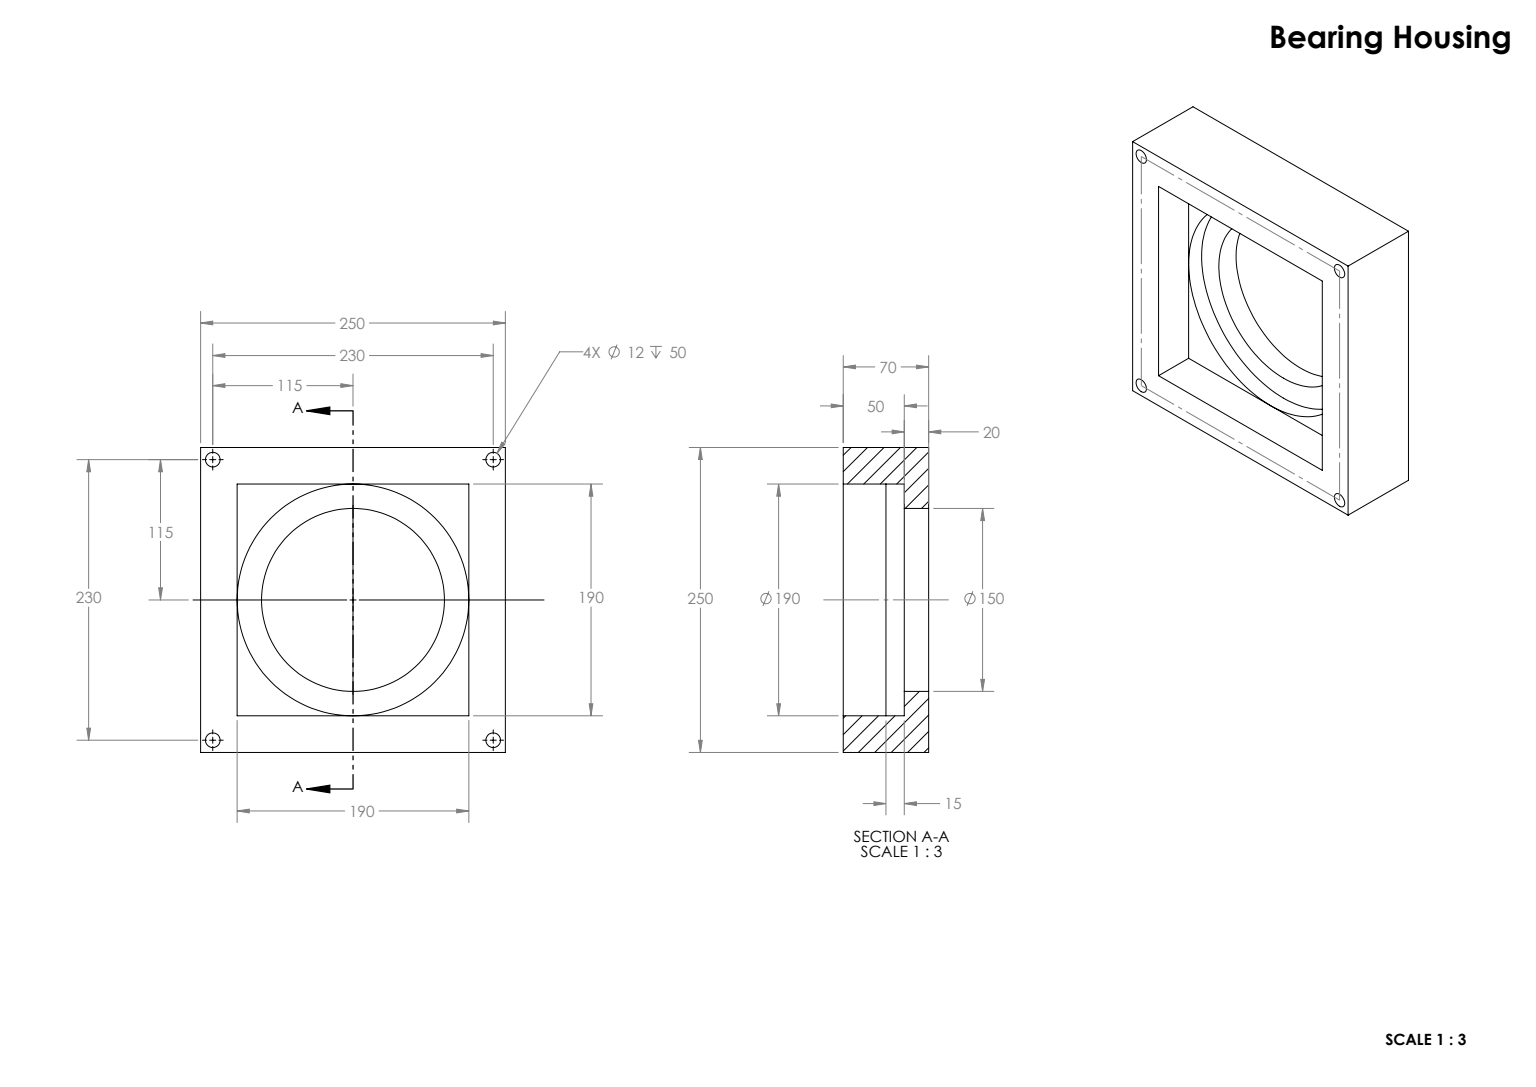
ISO-10303-21;
HEADER;
FILE_DESCRIPTION (('STEP AP214'),
    '1' );
FILE_NAME ('Bearing Housing.step',
    '2026-10-28T15:55:38',
    ( '' ),
    ( '' ),
    'SwSTEP 2.0',
    'SolidWorks 2025',
    '' );
FILE_SCHEMA (( 'AUTOMOTIVE_DESIGN' ));
ENDSEC;

DATA;
#4=LINE ( 'NONE', #7838, #2304 ) ;
#11=DIRECTION ( 'NONE',  ( 1.000000000000000000, 0.000000000000000000, 0.000000000000000000 ) ) ;
#20=DIRECTION ( 'NONE',  ( 0.000000000000000000, 0.000000000000000000, 1.000000000000000000 ) ) ;
#23=CARTESIAN_POINT ( 'NONE',  ( 0.000000000000000000, 0.000000000000000000, 20.00000000000000355 ) ) ;
#31=EDGE_CURVE ( 'NONE', #4444, #7082, #3495, .T. ) ;
#34=DIRECTION ( 'NONE',  ( -0.8571673007021112234, 1.049727191138617340E-16, 0.5150380749100560429 ) ) ;
#38=AXIS2_PLACEMENT_3D ( 'NONE', #602, #6938, #1699 ) ;
#44=ORIENTED_EDGE ( 'NONE', *, *, #3394, .T. ) ;
#47=AXIS2_PLACEMENT_3D ( 'NONE', #5788, #2622, #1664 ) ;
#52=ADVANCED_FACE ( 'NONE', ( #2135 ), #3528, .F. ) ;
#80=LINE ( 'NONE', #6946, #4020 ) ;
#96=ORIENTED_EDGE ( 'NONE', *, *, #4997, .F. ) ;
#128=DIRECTION ( 'NONE',  ( 1.000000000000000000, 0.000000000000000000, 0.000000000000000000 ) ) ;
#148=AXIS2_PLACEMENT_3D ( 'NONE', #811, #7440, #4371 ) ;
#150=ORIENTED_EDGE ( 'NONE', *, *, #4776, .F. ) ;
#160=CARTESIAN_POINT ( 'NONE',  ( -125.0000000000000000, -125.0000000000000284, 70.00000000000000000 ) ) ;
#167=VERTEX_POINT ( 'NONE', #2262 ) ;
#169=ORIENTED_EDGE ( 'NONE', *, *, #6813, .T. ) ;
#172=DIRECTION ( 'NONE',  ( 0.8571673007021112234, 0.000000000000000000, 0.5150380749100560429 ) ) ;
#194=LINE ( 'NONE', #930, #7129 ) ;
#195=DIRECTION ( 'NONE',  ( 0.8571673007021112234, 0.000000000000000000, 0.5150380749100560429 ) ) ;
#204=ADVANCED_FACE ( 'NONE', ( #6375 ), #5709, .F. ) ;
#215=VECTOR ( 'NONE', #34, 1000.000000000000000 ) ;
#226=EDGE_CURVE ( 'NONE', #3065, #4648, #8287, .T. ) ;
#228=DIRECTION ( 'NONE',  ( -0.000000000000000000, -0.000000000000000000, 1.000000000000000000 ) ) ;
#230=DIRECTION ( 'NONE',  ( 1.000000000000000000, 0.000000000000000000, 0.000000000000000000 ) ) ;
#251=DIRECTION ( 'NONE',  ( 1.000000000000000000, 0.000000000000000000, 0.000000000000000000 ) ) ;
#269=CARTESIAN_POINT ( 'NONE',  ( 121.0000000000000284, -115.0000000000000000, 20.00000000000000355 ) ) ;
#294=ORIENTED_EDGE ( 'NONE', *, *, #3089, .F. ) ;
#302=( NAMED_UNIT ( * ) SI_UNIT ( $, .STERADIAN. ) SOLID_ANGLE_UNIT ( ) );
#311=PLANE ( 'NONE',  #4412 ) ;
#313=DIRECTION ( 'NONE',  ( -0.000000000000000000, -0.000000000000000000, 1.000000000000000000 ) ) ;
#318=CARTESIAN_POINT ( 'NONE',  ( 115.0000000000000284, -115.0000000000000000, 20.00000000000000355 ) ) ;
#321=VERTEX_POINT ( 'NONE', #4199 ) ;
#324=CYLINDRICAL_SURFACE ( 'NONE', #1742, 5.999999999999991118 ) ;
#338=AXIS2_PLACEMENT_3D ( 'NONE', #4056, #6518, #5262 ) ;
#357=ORIENTED_EDGE ( 'NONE', *, *, #7077, .F. ) ;
#363=CARTESIAN_POINT ( 'NONE',  ( 115.0000000000000000, 115.0000000000000000, 70.00000000000000000 ) ) ;
#389=DIRECTION ( 'NONE',  ( -0.000000000000000000, -0.000000000000000000, 1.000000000000000000 ) ) ;
#390=AXIS2_PLACEMENT_3D ( 'NONE', #5966, #1418, #2752 ) ;
#393=ADVANCED_FACE ( 'NONE', ( #3838 ), #3197, .T. ) ;
#394=DIRECTION ( 'NONE',  ( 0.000000000000000000, 0.000000000000000000, 1.000000000000000000 ) ) ;
#396=EDGE_CURVE ( 'NONE', #4375, #2961, #3878, .T. ) ;
#398=DIRECTION ( 'NONE',  ( 0.000000000000000000, 0.000000000000000000, 1.000000000000000000 ) ) ;
#399=ORIENTED_EDGE ( 'NONE', *, *, #419, .F. ) ;
#400=LINE ( 'NONE', #8042, #670 ) ;
#405=ORIENTED_EDGE ( 'NONE', *, *, #8301, .F. ) ;
#409=ORIENTED_EDGE ( 'NONE', *, *, #5829, .F. ) ;
#410=FACE_OUTER_BOUND ( 'NONE', #2022, .T. ) ;
#419=EDGE_CURVE ( 'NONE', #3125, #7541, #3274, .T. ) ;
#421=VECTOR ( 'NONE', #7428, 1000.000000000000000 ) ;
#431=VERTEX_POINT ( 'NONE', #681 ) ;
#445=DIRECTION ( 'NONE',  ( 0.000000000000000000, 0.000000000000000000, 1.000000000000000000 ) ) ;
#451=DIRECTION ( 'NONE',  ( -1.000000000000000000, 0.000000000000000000, -0.000000000000000000 ) ) ;
#478=EDGE_LOOP ( 'NONE', ( #2078, #3169, #678, #44 ) ) ;
#481=ORIENTED_EDGE ( 'NONE', *, *, #4733, .F. ) ;
#485=EDGE_LOOP ( 'NONE', ( #1792, #6365 ) ) ;
#488=( GEOMETRIC_REPRESENTATION_CONTEXT ( 3 ) GLOBAL_UNCERTAINTY_ASSIGNED_CONTEXT ( ( #3697 ) ) GLOBAL_UNIT_ASSIGNED_CONTEXT ( ( #6897, #8033, #302 ) ) REPRESENTATION_CONTEXT ( 'NONE', 'WORKASPACE' ) );
#492=ORIENTED_EDGE ( 'NONE', *, *, #5575, .T. ) ;
#519=CONICAL_SURFACE ( 'NONE', #3466, 5.999999999999991118, 1.029744258676652313 ) ;
#520=LINE ( 'NONE', #6379, #1616 ) ;
#529=ADVANCED_FACE ( 'NONE', ( #545, #1858, #8136, #5692, #587, #3655 ), #2328, .F. ) ;
#530=EDGE_CURVE ( 'NONE', #7082, #2571, #3537, .T. ) ;
#545=FACE_BOUND ( 'NONE', #6221, .T. ) ;
#555=CARTESIAN_POINT ( 'NONE',  ( -94.99999999999997158, -95.00000000000008527, 35.00000000000000000 ) ) ;
#557=PRODUCT_DEFINITION ( 'UNKNOWN', '', #4198, #6779 ) ;
#560=ADVANCED_FACE ( 'NONE', ( #3064 ), #3869, .F. ) ;
#567=ORIENTED_EDGE ( 'NONE', *, *, #3332, .F. ) ;
#587=FACE_OUTER_BOUND ( 'NONE', #4365, .T. ) ;
#588=EDGE_LOOP ( 'NONE', ( #4360, #4935, #2316, #3157, #5452 ) ) ;
#590=DIRECTION ( 'NONE',  ( -0.000000000000000000, -0.000000000000000000, -1.000000000000000000 ) ) ;
#594=ADVANCED_BREP_SHAPE_REPRESENTATION ( '', ( #3512, #1299 ), #2770 ) ;
#599=ORIENTED_EDGE ( 'NONE', *, *, #1346, .F. ) ;
#602=CARTESIAN_POINT ( 'NONE',  ( 0.000000000000000000, 0.000000000000000000, 20.00000000000000355 ) ) ;
#606=ADVANCED_FACE ( 'NONE', ( #7629 ), #2357, .F. ) ;
#608=EDGE_LOOP ( 'NONE', ( #5995, #599, #5529 ) ) ;
#613=CARTESIAN_POINT ( 'NONE',  ( 0.000000000000000000, 0.000000000000000000, 35.00000000000000000 ) ) ;
#621=LINE ( 'NONE', #7198, #5046 ) ;
#631=ORIENTED_EDGE ( 'NONE', *, *, #7077, .T. ) ;
#635=DIRECTION ( 'NONE',  ( -0.000000000000000000, -0.000000000000000000, -1.000000000000000000 ) ) ;
#646=AXIS2_PLACEMENT_3D ( 'NONE', #788, #6612, #832 ) ;
#647=LINE ( 'NONE', #3893, #4845 ) ;
#663=DIRECTION ( 'NONE',  ( 1.000000000000000000, 0.000000000000000000, 0.000000000000000000 ) ) ;
#670=VECTOR ( 'NONE', #4828, 1000.000000000000000 ) ;
#673=CARTESIAN_POINT ( 'NONE',  ( 115.0000000000000284, -115.0000000000000000, 20.00000000000000355 ) ) ;
#675=DIRECTION ( 'NONE',  ( 0.000000000000000000, -1.000000000000000000, 0.000000000000000000 ) ) ;
#678=ORIENTED_EDGE ( 'NONE', *, *, #2723, .T. ) ;
#681=CARTESIAN_POINT ( 'NONE',  ( 95.00000000000000000, 95.00000000000008527, 35.00000000000000000 ) ) ;
#682=LINE ( 'NONE', #2005, #3999 ) ;
#704=DIRECTION ( 'NONE',  ( -0.000000000000000000, -0.000000000000000000, -1.000000000000000000 ) ) ;
#709=CARTESIAN_POINT ( 'NONE',  ( 0.000000000000000000, 0.000000000000000000, 35.00000000000000000 ) ) ;
#738=VECTOR ( 'NONE', #3922, 1000.000000000000000 ) ;
#749=FACE_OUTER_BOUND ( 'NONE', #4846, .T. ) ;
#750=ORIENTED_EDGE ( 'NONE', *, *, #3807, .F. ) ;
#761=CARTESIAN_POINT ( 'NONE',  ( -121.0000000000000284, -115.0000000000000000, 70.00000000000000000 ) ) ;
#765=CIRCLE ( 'NONE', #5482, 5.999999999999991118 ) ;
#770=DIRECTION ( 'NONE',  ( -0.8571673007021112234, 1.049727191138617340E-16, 0.5150380749100560429 ) ) ;
#783=VECTOR ( 'NONE', #770, 1000.000000000000000 ) ;
#784=LINE ( 'NONE', #7845, #3091 ) ;
#788=CARTESIAN_POINT ( 'NONE',  ( -125.0000000000000000, -125.0000000000000284, 70.00000000000000000 ) ) ;
#811=CARTESIAN_POINT ( 'NONE',  ( -115.0000000000000000, 115.0000000000000000, 70.00000000000000000 ) ) ;
#824=ADVANCED_FACE ( 'NONE', ( #6135 ), #881, .F. ) ;
#832=DIRECTION ( 'NONE',  ( 0.000000000000000000, 0.000000000000000000, -1.000000000000000000 ) ) ;
#840=EDGE_CURVE ( 'NONE', #4413, #3125, #621, .T. ) ;
#845=ORIENTED_EDGE ( 'NONE', *, *, #5575, .F. ) ;
#858=AXIS2_PLACEMENT_3D ( 'NONE', #1793, #3675, #1748 ) ;
#865=CARTESIAN_POINT ( 'NONE',  ( -125.0000000000000000, 125.0000000000000284, 70.00000000000000000 ) ) ;
#867=CARTESIAN_POINT ( 'NONE',  ( 125.0000000000000000, -125.0000000000000284, 70.00000000000000000 ) ) ;
#868=LINE ( 'NONE', #4741, #4236 ) ;
#881=CYLINDRICAL_SURFACE ( 'NONE', #5727, 95.00000000000008527 ) ;
#887=ORIENTED_EDGE ( 'NONE', *, *, #4997, .T. ) ;
#894=DIRECTION ( 'NONE',  ( 0.000000000000000000, -0.000000000000000000, -1.000000000000000000 ) ) ;
#899=ORIENTED_EDGE ( 'NONE', *, *, #2632, .F. ) ;
#904=CARTESIAN_POINT ( 'NONE',  ( 121.0000000000000284, -115.0000000000000000, 20.00000000000000355 ) ) ;
#910=FACE_OUTER_BOUND ( 'NONE', #7824, .T. ) ;
#930=CARTESIAN_POINT ( 'NONE',  ( -94.99999999999997158, -95.00000000000008527, 70.00000000000000000 ) ) ;
#946=EDGE_LOOP ( 'NONE', ( #1027, #5506, #399, #5076 ) ) ;
#948=FACE_OUTER_BOUND ( 'NONE', #4156, .T. ) ;
#984=VERTEX_POINT ( 'NONE', #1023 ) ;
#985=CARTESIAN_POINT ( 'NONE',  ( -115.0000000000000000, 115.0000000000000000, 20.00000000000000355 ) ) ;
#999=DIRECTION ( 'NONE',  ( -1.000000000000000000, -2.921639538487254261E-16, 0.000000000000000000 ) ) ;
#1002=DIRECTION ( 'NONE',  ( 1.000000000000000000, 0.000000000000000000, 0.000000000000000000 ) ) ;
#1003=ORIENTED_EDGE ( 'NONE', *, *, #8301, .T. ) ;
#1015=EDGE_CURVE ( 'NONE', #7541, #321, #4599, .T. ) ;
#1023=CARTESIAN_POINT ( 'NONE',  ( 0.000000000000000000, 95.00000000000008527, 35.00000000000000000 ) ) ;
#1027=ORIENTED_EDGE ( 'NONE', *, *, #7821, .F. ) ;
#1030=VECTOR ( 'NONE', #5810, 1000.000000000000000 ) ;
#1045=FACE_OUTER_BOUND ( 'NONE', #5118, .T. ) ;
#1071=CARTESIAN_POINT ( 'NONE',  ( 115.0000000000000142, -115.0000000000000000, 16.39483628583463570 ) ) ;
#1074=DIRECTION ( 'NONE',  ( 0.000000000000000000, 0.000000000000000000, 1.000000000000000000 ) ) ;
#1085=LINE ( 'NONE', #1631, #4556 ) ;
#1086=CIRCLE ( 'NONE', #5804, 5.999999999999991118 ) ;
#1090=DIRECTION ( 'NONE',  ( -0.000000000000000000, -0.000000000000000000, 1.000000000000000000 ) ) ;
#1096=ORIENTED_EDGE ( 'NONE', *, *, #5028, .T. ) ;
#1097=CARTESIAN_POINT ( 'NONE',  ( -109.0000000000000426, -115.0000000000000000, 20.00000000000000355 ) ) ;
#1102=ORIENTED_EDGE ( 'NONE', *, *, #8208, .F. ) ;
#1111=CARTESIAN_POINT ( 'NONE',  ( -95.00000000000008527, 1.163414459189986590E-14, 20.00000000000000355 ) ) ;
#1137=EDGE_LOOP ( 'NONE', ( #6698, #6760, #1494 ) ) ;
#1140=ORIENTED_EDGE ( 'NONE', *, *, #7652, .T. ) ;
#1142=DIRECTION ( 'NONE',  ( -0.000000000000000000, -0.000000000000000000, 1.000000000000000000 ) ) ;
#1162=LINE ( 'NONE', #2390, #1897 ) ;
#1173=CIRCLE ( 'NONE', #5753, 5.999999999999991118 ) ;
#1182=FACE_OUTER_BOUND ( 'NONE', #1137, .T. ) ;
#1188=EDGE_CURVE ( 'NONE', #4648, #3065, #3811, .T. ) ;
#1194=DIRECTION ( 'NONE',  ( -0.000000000000000000, -0.000000000000000000, 1.000000000000000000 ) ) ;
#1197=EDGE_CURVE ( 'NONE', #4172, #3595, #4328, .T. ) ;
#1226=DIRECTION ( 'NONE',  ( -0.000000000000000000, -0.000000000000000000, 1.000000000000000000 ) ) ;
#1227=PLANE ( 'NONE',  #7361 ) ;
#1245=EDGE_CURVE ( 'NONE', #6477, #2906, #6366, .T. ) ;
#1253=DIRECTION ( 'NONE',  ( 0.000000000000000000, 0.000000000000000000, -1.000000000000000000 ) ) ;
#1267=FACE_OUTER_BOUND ( 'NONE', #4745, .T. ) ;
#1276=VECTOR ( 'NONE', #1311, 1000.000000000000000 ) ;
#1277=VERTEX_POINT ( 'NONE', #7565 ) ;
#1280=DIRECTION ( 'NONE',  ( -0.000000000000000000, -0.000000000000000000, 1.000000000000000000 ) ) ;
#1286=EDGE_LOOP ( 'NONE', ( #1102, #7331, #2428 ) ) ;
#1287=ORIENTED_EDGE ( 'NONE', *, *, #6688, .F. ) ;
#1290=DIRECTION ( 'NONE',  ( -0.000000000000000000, -0.000000000000000000, 1.000000000000000000 ) ) ;
#1293=CARTESIAN_POINT ( 'NONE',  ( -115.0000000000000000, 115.0000000000000000, 70.00000000000000000 ) ) ;
#1299=AXIS2_PLACEMENT_3D ( 'NONE', #5884, #1507, #5927 ) ;
#1310=ORIENTED_EDGE ( 'NONE', *, *, #2278, .T. ) ;
#1311=DIRECTION ( 'NONE',  ( 1.000000000000000000, -0.000000000000000000, -0.000000000000000000 ) ) ;
#1346=EDGE_CURVE ( 'NONE', #4671, #5876, #4609, .T. ) ;
#1371=DIRECTION ( 'NONE',  ( -1.000000000000000000, -2.921639538487254261E-16, 0.000000000000000000 ) ) ;
#1389=LINE ( 'NONE', #5624, #1594 ) ;
#1396=ORIENTED_EDGE ( 'NONE', *, *, #3184, .T. ) ;
#1409=DIRECTION ( 'NONE',  ( -0.000000000000000000, -0.000000000000000000, 1.000000000000000000 ) ) ;
#1414=ORIENTED_EDGE ( 'NONE', *, *, #8095, .F. ) ;
#1418=DIRECTION ( 'NONE',  ( -0.000000000000000000, -0.000000000000000000, 1.000000000000000000 ) ) ;
#1421=FACE_OUTER_BOUND ( 'NONE', #1500, .T. ) ;
#1423=DIRECTION ( 'NONE',  ( 1.000000000000000000, 0.000000000000000000, 0.000000000000000000 ) ) ;
#1452=ORIENTED_EDGE ( 'NONE', *, *, #5795, .T. ) ;
#1455=CARTESIAN_POINT ( 'NONE',  ( 95.00000000000008527, 1.387778780781445991E-14, 35.00000000000000000 ) ) ;
#1456=ADVANCED_FACE ( 'NONE', ( #910 ), #8038, .F. ) ;
#1466=DIRECTION ( 'NONE',  ( 1.000000000000000000, 0.000000000000000000, 0.000000000000000000 ) ) ;
#1478=EDGE_LOOP ( 'NONE', ( #2814, #4335, #7683, #8119 ) ) ;
#1484=EDGE_CURVE ( 'NONE', #6102, #3725, #5831, .T. ) ;
#1494=ORIENTED_EDGE ( 'NONE', *, *, #530, .T. ) ;
#1497=ADVANCED_FACE ( 'NONE', ( #5339 ), #2472, .F. ) ;
#1500=EDGE_LOOP ( 'NONE', ( #2987, #3974, #150, #5372 ) ) ;
#1507=DIRECTION ( 'NONE',  ( 0.000000000000000000, 0.000000000000000000, 1.000000000000000000 ) ) ;
#1509=LINE ( 'NONE', #4179, #8200 ) ;
#1517=CARTESIAN_POINT ( 'NONE',  ( 115.0000000000000284, -115.0000000000000000, 70.00000000000000000 ) ) ;
#1526=CARTESIAN_POINT ( 'NONE',  ( 0.000000000000000000, 0.000000000000000000, 20.00000000000000355 ) ) ;
#1528=DIRECTION ( 'NONE',  ( 0.000000000000000000, 0.000000000000000000, -1.000000000000000000 ) ) ;
#1561=CARTESIAN_POINT ( 'NONE',  ( 109.0000000000000426, -115.0000000000000000, 70.00000000000000000 ) ) ;
#1564=EDGE_CURVE ( 'NONE', #2906, #6477, #2478, .T. ) ;
#1569=VECTOR ( 'NONE', #8345, 1000.000000000000000 ) ;
#1570=LINE ( 'NONE', #160, #5897 ) ;
#1577=ORIENTED_EDGE ( 'NONE', *, *, #2769, .T. ) ;
#1583=CIRCLE ( 'NONE', #5077, 75.00000000000001421 ) ;
#1594=VECTOR ( 'NONE', #7128, 1000.000000000000000 ) ;
#1600=ADVANCED_FACE ( 'NONE', ( #3544, #6125 ), #5512, .T. ) ;
#1616=VECTOR ( 'NONE', #7534, 1000.000000000000000 ) ;
#1631=CARTESIAN_POINT ( 'NONE',  ( 95.00000000000002842, -95.00000000000002842, 35.00000000000000000 ) ) ;
#1639=CIRCLE ( 'NONE', #6351, 75.00000000000001421 ) ;
#1664=DIRECTION ( 'NONE',  ( -1.000000000000000000, -2.921639538487254261E-16, 0.000000000000000000 ) ) ;
#1667=CLOSED_SHELL ( 'NONE', ( #2679, #1880, #7336, #2122, #6642, #3883, #8031, #3707, #824, #6804, #606, #5668, #52, #4927, #1815, #5762, #393, #2091, #529, #4372, #8145, #2776, #6343, #204, #3859, #1600, #7114, #6811, #2441, #3318, #560, #4099, #1456, #1497, #6513 ) ) ;
#1668=CARTESIAN_POINT ( 'NONE',  ( -94.99999999999997158, -95.00000000000008527, 70.00000000000000000 ) ) ;
#1670=DIRECTION ( 'NONE',  ( 0.000000000000000000, 0.000000000000000000, -1.000000000000000000 ) ) ;
#1684=ORIENTED_EDGE ( 'NONE', *, *, #2388, .T. ) ;
#1699=DIRECTION ( 'NONE',  ( 1.000000000000000000, 0.000000000000000000, 0.000000000000000000 ) ) ;
#1734=ORIENTED_EDGE ( 'NONE', *, *, #5795, .F. ) ;
#1735=DIRECTION ( 'NONE',  ( -0.000000000000000000, -0.000000000000000000, -1.000000000000000000 ) ) ;
#1742=AXIS2_PLACEMENT_3D ( 'NONE', #2367, #4918, #4885 ) ;
#1748=DIRECTION ( 'NONE',  ( 0.000000000000000000, 0.000000000000000000, 1.000000000000000000 ) ) ;
#1763=CARTESIAN_POINT ( 'NONE',  ( -115.0000000000000000, 115.0000000000000000, 70.00000000000000000 ) ) ;
#1766=VECTOR ( 'NONE', #3795, 1000.000000000000000 ) ;
#1768=ORIENTED_EDGE ( 'NONE', *, *, #4192, .T. ) ;
#1773=ORIENTED_EDGE ( 'NONE', *, *, #396, .T. ) ;
#1783=EDGE_LOOP ( 'NONE', ( #8289, #4269, #7405, #2363 ) ) ;
#1785=CYLINDRICAL_SURFACE ( 'NONE', #1873, 75.00000000000001421 ) ;
#1792=ORIENTED_EDGE ( 'NONE', *, *, #3763, .F. ) ;
#1793=CARTESIAN_POINT ( 'NONE',  ( 125.0000000000000000, -125.0000000000000284, 70.00000000000000000 ) ) ;
#1802=CARTESIAN_POINT ( 'NONE',  ( 95.00000000000000000, 95.00000000000008527, 70.00000000000000000 ) ) ;
#1815=ADVANCED_FACE ( 'NONE', ( #7307 ), #4081, .T. ) ;
#1820=EDGE_LOOP ( 'NONE', ( #4840, #1734, #409 ) ) ;
#1850=LINE ( 'NONE', #2451, #2663 ) ;
#1852=ORIENTED_EDGE ( 'NONE', *, *, #7492, .T. ) ;
#1854=AXIS2_PLACEMENT_3D ( 'NONE', #4858, #5664, #6078 ) ;
#1858=FACE_BOUND ( 'NONE', #485, .T. ) ;
#1866=EDGE_CURVE ( 'NONE', #6494, #167, #4693, .T. ) ;
#1873=AXIS2_PLACEMENT_3D ( 'NONE', #7567, #1735, #7517 ) ;
#1880=ADVANCED_FACE ( 'NONE', ( #948 ), #2153, .F. ) ;
#1897=VECTOR ( 'NONE', #1280, 1000.000000000000000 ) ;
#1906=ORIENTED_EDGE ( 'NONE', *, *, #2484, .T. ) ;
#1940=CARTESIAN_POINT ( 'NONE',  ( 115.0000000000000284, -115.0000000000000000, 70.00000000000000000 ) ) ;
#1949=ORIENTED_EDGE ( 'NONE', *, *, #8105, .F. ) ;
#1979=FACE_OUTER_BOUND ( 'NONE', #608, .T. ) ;
#1994=ORIENTED_EDGE ( 'NONE', *, *, #2474, .T. ) ;
#2003=MECHANICAL_DESIGN_GEOMETRIC_PRESENTATION_REPRESENTATION('',(#5880),#488);
#2005=CARTESIAN_POINT ( 'NONE',  ( 121.0000000000000284, -115.0000000000000000, 70.00000000000000000 ) ) ;
#2010=AXIS2_PLACEMENT_3D ( 'NONE', #7360, #7954, #8028 ) ;
#2015=CARTESIAN_POINT ( 'NONE',  ( 95.00000000000002842, -95.00000000000002842, 70.00000000000000000 ) ) ;
#2022=EDGE_LOOP ( 'NONE', ( #6636, #1140, #3559, #3514 ) ) ;
#2052=ORIENTED_EDGE ( 'NONE', *, *, #6603, .T. ) ;
#2064=PRODUCT_DEFINITION_SHAPE ( 'NONE', 'NONE',  #557 ) ;
#2078=ORIENTED_EDGE ( 'NONE', *, *, #8225, .F. ) ;
#2085=AXIS2_PLACEMENT_3D ( 'NONE', #5602, #445, #663 ) ;
#2091=ADVANCED_FACE ( 'NONE', ( #2215 ), #6199, .T. ) ;
#2093=CARTESIAN_POINT ( 'NONE',  ( 125.0000000000000000, -125.0000000000000284, 70.00000000000000000 ) ) ;
#2107=ORIENTED_EDGE ( 'NONE', *, *, #1564, .T. ) ;
#2122=ADVANCED_FACE ( 'NONE', ( #6834 ), #5407, .F. ) ;
#2135=FACE_OUTER_BOUND ( 'NONE', #1820, .T. ) ;
#2147=SHAPE_REPRESENTATION_RELATIONSHIP ( 'NONE' , 'NONE' ,  #2264, #594 ) ;
#2153=CONICAL_SURFACE ( 'NONE', #6444, 5.999999999999991118, 1.029744258676652313 ) ;
#2159=VECTOR ( 'NONE', #4968, 1000.000000000000000 ) ;
#2161=ORIENTED_EDGE ( 'NONE', *, *, #3332, .T. ) ;
#2165=ORIENTED_EDGE ( 'NONE', *, *, #1564, .F. ) ;
#2181=CARTESIAN_POINT ( 'NONE',  ( 115.0000000000000284, -115.0000000000000000, 20.00000000000000355 ) ) ;
#2183=EDGE_CURVE ( 'NONE', #2571, #5439, #5014, .T. ) ;
#2205=LINE ( 'NONE', #5561, #421 ) ;
#2208=UNCERTAINTY_MEASURE_WITH_UNIT (LENGTH_MEASURE( 1.000000000000000082E-05 ), #5967, 'distance_accuracy_value', 'NONE');
#2212=CYLINDRICAL_SURFACE ( 'NONE', #3779, 5.999999999999991118 ) ;
#2215=FACE_OUTER_BOUND ( 'NONE', #4169, .T. ) ;
#2221=LINE ( 'NONE', #4002, #783 ) ;
#2243=CARTESIAN_POINT ( 'NONE',  ( 0.000000000000000000, 0.000000000000000000, 35.00000000000000000 ) ) ;
#2258=ORIENTED_EDGE ( 'NONE', *, *, #2769, .F. ) ;
#2262=CARTESIAN_POINT ( 'NONE',  ( -109.0000000000000426, -115.0000000000000000, 70.00000000000000000 ) ) ;
#2264=SHAPE_REPRESENTATION ( 'Bearing Housing', ( #1299 ), #2770 ) ;
#2266=AXIS2_PLACEMENT_3D ( 'NONE', #613, #1253, #7661 ) ;
#2278=EDGE_CURVE ( 'NONE', #3595, #167, #7171, .T. ) ;
#2295=DIRECTION ( 'NONE',  ( 1.460819769243626145E-16, -1.000000000000000000, 0.000000000000000000 ) ) ;
#2304=VECTOR ( 'NONE', #7793, 1000.000000000000000 ) ;
#2313=DIRECTION ( 'NONE',  ( 1.000000000000000000, 0.000000000000000000, -0.000000000000000000 ) ) ;
#2316=ORIENTED_EDGE ( 'NONE', *, *, #7896, .T. ) ;
#2317=FACE_OUTER_BOUND ( 'NONE', #4232, .T. ) ;
#2318=DIRECTION ( 'NONE',  ( 1.000000000000000000, 0.000000000000000000, 0.000000000000000000 ) ) ;
#2328=PLANE ( 'NONE',  #7482 ) ;
#2340=DIRECTION ( 'NONE',  ( -0.000000000000000000, -0.000000000000000000, 1.000000000000000000 ) ) ;
#2341=AXIS2_PLACEMENT_3D ( 'NONE', #1763, #7458, #3682 ) ;
#2344=ORIENTED_EDGE ( 'NONE', *, *, #7429, .F. ) ;
#2357=PLANE ( 'NONE',  #2368 ) ;
#2360=DIRECTION ( 'NONE',  ( -0.000000000000000000, -0.000000000000000000, 1.000000000000000000 ) ) ;
#2363=ORIENTED_EDGE ( 'NONE', *, *, #5060, .T. ) ;
#2367=CARTESIAN_POINT ( 'NONE',  ( -115.0000000000000284, -115.0000000000000000, 70.00000000000000000 ) ) ;
#2368=AXIS2_PLACEMENT_3D ( 'NONE', #2922, #1670, #8264 ) ;
#2388=EDGE_CURVE ( 'NONE', #7988, #7828, #2205, .T. ) ;
#2390=CARTESIAN_POINT ( 'NONE',  ( -121.0000000000000284, -115.0000000000000000, 70.00000000000000000 ) ) ;
#2400=EDGE_LOOP ( 'NONE', ( #4395, #3990 ) ) ;
#2402=DIRECTION ( 'NONE',  ( -0.000000000000000000, -0.000000000000000000, 1.000000000000000000 ) ) ;
#2428=ORIENTED_EDGE ( 'NONE', *, *, #1484, .T. ) ;
#2439=ORIENTED_EDGE ( 'NONE', *, *, #7821, .T. ) ;
#2441=ADVANCED_FACE ( 'NONE', ( #1045 ), #7338, .F. ) ;
#2443=CARTESIAN_POINT ( 'NONE',  ( -94.99999999999997158, -95.00000000000008527, 35.00000000000000000 ) ) ;
#2447=CARTESIAN_POINT ( 'NONE',  ( 109.0000000000000142, 115.0000000000000000, 70.00000000000000000 ) ) ;
#2451=CARTESIAN_POINT ( 'NONE',  ( 95.00000000000002842, -95.00000000000002842, 70.00000000000000000 ) ) ;
#2459=DIRECTION ( 'NONE',  ( -0.000000000000000000, -0.000000000000000000, 1.000000000000000000 ) ) ;
#2469=EDGE_LOOP ( 'NONE', ( #2258, #6415 ) ) ;
#2472=CONICAL_SURFACE ( 'NONE', #3513, 5.999999999999991118, 1.029744258676652313 ) ;
#2474=EDGE_CURVE ( 'NONE', #2571, #7082, #3245, .T. ) ;
#2478=CIRCLE ( 'NONE', #2341, 5.999999999999991118 ) ;
#2484=EDGE_CURVE ( 'NONE', #5937, #3656, #1639, .T. ) ;
#2489=CARTESIAN_POINT ( 'NONE',  ( 109.0000000000000426, -115.0000000000000000, 20.00000000000000355 ) ) ;
#2494=CARTESIAN_POINT ( 'NONE',  ( 0.000000000000000000, 0.000000000000000000, 70.00000000000000000 ) ) ;
#2497=DIRECTION ( 'NONE',  ( -0.000000000000000000, -0.000000000000000000, 1.000000000000000000 ) ) ;
#2499=PRODUCT_CONTEXT ( 'NONE', #5106, 'mechanical' ) ;
#2516=VECTOR ( 'NONE', #6500, 1000.000000000000000 ) ;
#2530=CONICAL_SURFACE ( 'NONE', #3578, 5.999999999999991118, 1.029744258676652313 ) ;
#2547=ORIENTED_EDGE ( 'NONE', *, *, #5060, .F. ) ;
#2553=AXIS2_PLACEMENT_3D ( 'NONE', #709, #3266, #5935 ) ;
#2566=DIRECTION ( 'NONE',  ( -0.000000000000000000, -1.000000000000000000, -0.000000000000000000 ) ) ;
#2571=VERTEX_POINT ( 'NONE', #2489 ) ;
#2589=EDGE_LOOP ( 'NONE', ( #7615, #4290, #6395, #5202 ) ) ;
#2592=ORIENTED_EDGE ( 'NONE', *, *, #2183, .T. ) ;
#2593=AXIS2_PLACEMENT_3D ( 'NONE', #1517, #6742, #230 ) ;
#2611=ORIENTED_EDGE ( 'NONE', *, *, #6278, .T. ) ;
#2612=VERTEX_POINT ( 'NONE', #3108 ) ;
#2622=DIRECTION ( 'NONE',  ( -2.921639538487254261E-16, 1.000000000000000000, 0.000000000000000000 ) ) ;
#2632=EDGE_CURVE ( 'NONE', #7988, #3069, #1850, .T. ) ;
#2659=VECTOR ( 'NONE', #195, 1000.000000000000000 ) ;
#2663=VECTOR ( 'NONE', #3824, 1000.000000000000000 ) ;
#2671=CARTESIAN_POINT ( 'NONE',  ( 75.00000000000001421, 9.184850993605150311E-15, 20.00000000000000355 ) ) ;
#2679=ADVANCED_FACE ( 'NONE', ( #4914 ), #6867, .F. ) ;
#2684=FACE_OUTER_BOUND ( 'NONE', #4430, .T. ) ;
#2687=DIRECTION ( 'NONE',  ( -0.000000000000000000, -0.000000000000000000, 1.000000000000000000 ) ) ;
#2689=ORIENTED_EDGE ( 'NONE', *, *, #7492, .F. ) ;
#2723=EDGE_CURVE ( 'NONE', #3656, #5338, #5303, .T. ) ;
#2752=DIRECTION ( 'NONE',  ( 1.000000000000000000, 0.000000000000000000, 0.000000000000000000 ) ) ;
#2754=DIRECTION ( 'NONE',  ( -1.460819769243625652E-16, 1.000000000000000000, 0.000000000000000000 ) ) ;
#2769=EDGE_CURVE ( 'NONE', #167, #6494, #2792, .T. ) ;
#2770=( GEOMETRIC_REPRESENTATION_CONTEXT ( 3 ) GLOBAL_UNCERTAINTY_ASSIGNED_CONTEXT ( ( #2208 ) ) GLOBAL_UNIT_ASSIGNED_CONTEXT ( ( #5967, #3298, #4614 ) ) REPRESENTATION_CONTEXT ( 'NONE', 'WORKASPACE' ) );
#2774=AXIS2_PLACEMENT_3D ( 'NONE', #2181, #1409, #4730 ) ;
#2776=ADVANCED_FACE ( 'NONE', ( #1421 ), #6566, .F. ) ;
#2792=CIRCLE ( 'NONE', #4539, 5.999999999999991118 ) ;
#2793=FACE_OUTER_BOUND ( 'NONE', #946, .T. ) ;
#2802=CARTESIAN_POINT ( 'NONE',  ( -115.0000000000000142, 115.0000000000000000, 16.39483628583463570 ) ) ;
#2814=ORIENTED_EDGE ( 'NONE', *, *, #2484, .F. ) ;
#2815=EDGE_CURVE ( 'NONE', #2961, #321, #1509, .T. ) ;
#2816=FACE_OUTER_BOUND ( 'NONE', #3661, .T. ) ;
#2831=ORIENTED_EDGE ( 'NONE', *, *, #6813, .F. ) ;
#2833=ORIENTED_EDGE ( 'NONE', *, *, #8208, .T. ) ;
#2849=AXIS2_PLACEMENT_3D ( 'NONE', #5425, #7291, #1466 ) ;
#2854=LINE ( 'NONE', #1097, #2159 ) ;
#2885=DIRECTION ( 'NONE',  ( 1.000000000000000000, 0.000000000000000000, 0.000000000000000000 ) ) ;
#2904=CIRCLE ( 'NONE', #5747, 5.999999999999991118 ) ;
#2906=VERTEX_POINT ( 'NONE', #6731 ) ;
#2908=VECTOR ( 'NONE', #8122, 1000.000000000000000 ) ;
#2922=CARTESIAN_POINT ( 'NONE',  ( 0.000000000000000000, 0.000000000000000000, 35.00000000000000000 ) ) ;
#2927=LINE ( 'NONE', #5519, #4384 ) ;
#2928=ORIENTED_EDGE ( 'NONE', *, *, #2183, .F. ) ;
#2937=AXIS2_PLACEMENT_3D ( 'NONE', #7638, #4399, #5778 ) ;
#2951=AXIS2_PLACEMENT_3D ( 'NONE', #8328, #7050, #5827 ) ;
#2961=VERTEX_POINT ( 'NONE', #7273 ) ;
#2986=CARTESIAN_POINT ( 'NONE',  ( 115.0000000000000000, 115.0000000000000000, 20.00000000000000355 ) ) ;
#2987=ORIENTED_EDGE ( 'NONE', *, *, #840, .T. ) ;
#3032=ORIENTED_EDGE ( 'NONE', *, *, #3319, .F. ) ;
#3049=CARTESIAN_POINT ( 'NONE',  ( -109.0000000000000142, 115.0000000000000000, 20.00000000000000355 ) ) ;
#3064=FACE_OUTER_BOUND ( 'NONE', #4958, .T. ) ;
#3065=VERTEX_POINT ( 'NONE', #1111 ) ;
#3067=FACE_OUTER_BOUND ( 'NONE', #5317, .T. ) ;
#3069=VERTEX_POINT ( 'NONE', #6440 ) ;
#3081=ORIENTED_EDGE ( 'NONE', *, *, #3910, .F. ) ;
#3084=DIRECTION ( 'NONE',  ( -1.000000000000000000, 0.000000000000000000, 0.000000000000000000 ) ) ;
#3089=EDGE_CURVE ( 'NONE', #5894, #5749, #1389, .T. ) ;
#3091=VECTOR ( 'NONE', #3374, 1000.000000000000000 ) ;
#3108=CARTESIAN_POINT ( 'NONE',  ( -95.00000000000000000, 95.00000000000008527, 70.00000000000000000 ) ) ;
#3109=ORIENTED_EDGE ( 'NONE', *, *, #4431, .F. ) ;
#3125=VERTEX_POINT ( 'NONE', #6009 ) ;
#3157=ORIENTED_EDGE ( 'NONE', *, *, #3184, .F. ) ;
#3169=ORIENTED_EDGE ( 'NONE', *, *, #8157, .F. ) ;
#3182=CONICAL_SURFACE ( 'NONE', #1854, 5.999999999999991118, 1.029744258676652313 ) ;
#3184=EDGE_CURVE ( 'NONE', #7934, #6392, #3386, .T. ) ;
#3197=PLANE ( 'NONE',  #47 ) ;
#3204=CARTESIAN_POINT ( 'NONE',  ( -121.0000000000000284, -115.0000000000000000, 20.00000000000000355 ) ) ;
#3211=CARTESIAN_POINT ( 'NONE',  ( -109.0000000000000426, -115.0000000000000000, 20.00000000000000355 ) ) ;
#3214=VECTOR ( 'NONE', #3821, 1000.000000000000000 ) ;
#3216=LINE ( 'NONE', #7674, #6696 ) ;
#3217=LINE ( 'NONE', #4351, #3214 ) ;
#3230=DIRECTION ( 'NONE',  ( 1.000000000000000000, 0.000000000000000000, 0.000000000000000000 ) ) ;
#3233=DIRECTION ( 'NONE',  ( 1.000000000000000000, 0.000000000000000000, 0.000000000000000000 ) ) ;
#3245=CIRCLE ( 'NONE', #5948, 5.999999999999991118 ) ;
#3256=DIRECTION ( 'NONE',  ( -0.000000000000000000, -0.000000000000000000, 1.000000000000000000 ) ) ;
#3257=CARTESIAN_POINT ( 'NONE',  ( -95.00000000000000000, 95.00000000000008527, 35.00000000000000000 ) ) ;
#3266=DIRECTION ( 'NONE',  ( 0.000000000000000000, 0.000000000000000000, -1.000000000000000000 ) ) ;
#3272=VECTOR ( 'NONE', #172, 1000.000000000000000 ) ;
#3274=LINE ( 'NONE', #5145, #1276 ) ;
#3285=CARTESIAN_POINT ( 'NONE',  ( -94.99999999999998579, -1.387778780781444098E-14, 35.00000000000000000 ) ) ;
#3298=( NAMED_UNIT ( * ) PLANE_ANGLE_UNIT ( ) SI_UNIT ( $, .RADIAN. ) );
#3318=ADVANCED_FACE ( 'NONE', ( #6183 ), #6687, .F. ) ;
#3319=EDGE_CURVE ( 'NONE', #4648, #4314, #2927, .T. ) ;
#3326=CARTESIAN_POINT ( 'NONE',  ( -94.99999999999997158, -95.00000000000008527, 70.00000000000000000 ) ) ;
#3332=EDGE_CURVE ( 'NONE', #3595, #4172, #765, .T. ) ;
#3333=EDGE_CURVE ( 'NONE', #6102, #8341, #4871, .T. ) ;
#3374=DIRECTION ( 'NONE',  ( -0.000000000000000000, -0.000000000000000000, 1.000000000000000000 ) ) ;
#3375=EDGE_CURVE ( 'NONE', #5439, #5603, #2904, .T. ) ;
#3386=LINE ( 'NONE', #7297, #4260 ) ;
#3394=EDGE_CURVE ( 'NONE', #5338, #6480, #7645, .T. ) ;
#3402=CARTESIAN_POINT ( 'NONE',  ( -109.0000000000000142, 115.0000000000000000, 70.00000000000000000 ) ) ;
#3426=CARTESIAN_POINT ( 'NONE',  ( 0.000000000000000000, 0.000000000000000000, 20.00000000000000355 ) ) ;
#3428=EDGE_CURVE ( 'NONE', #5586, #4375, #6609, .T. ) ;
#3438=DIRECTION ( 'NONE',  ( 1.000000000000000000, 0.000000000000000000, 0.000000000000000000 ) ) ;
#3452=VECTOR ( 'NONE', #7869, 1000.000000000000000 ) ;
#3461=CARTESIAN_POINT ( 'NONE',  ( 115.0000000000000000, 115.0000000000000000, 70.00000000000000000 ) ) ;
#3466=AXIS2_PLACEMENT_3D ( 'NONE', #673, #1226, #3230 ) ;
#3488=DIRECTION ( 'NONE',  ( 1.000000000000000000, 0.000000000000000000, 0.000000000000000000 ) ) ;
#3492=ORIENTED_EDGE ( 'NONE', *, *, #4092, .F. ) ;
#3495=LINE ( 'NONE', #904, #3272 ) ;
#3496=CARTESIAN_POINT ( 'NONE',  ( 0.000000000000000000, 0.000000000000000000, 35.00000000000000000 ) ) ;
#3503=DIRECTION ( 'NONE',  ( -0.000000000000000000, -0.000000000000000000, 1.000000000000000000 ) ) ;
#3505=CARTESIAN_POINT ( 'NONE',  ( -115.0000000000000284, -115.0000000000000000, 70.00000000000000000 ) ) ;
#3512=MANIFOLD_SOLID_BREP ( '\X2\00d8\X0\12.0mm Dowel Hole1', #1667 ) ;
#3513=AXIS2_PLACEMENT_3D ( 'NONE', #5385, #3503, #7964 ) ;
#3514=ORIENTED_EDGE ( 'NONE', *, *, #2278, .F. ) ;
#3519=ORIENTED_EDGE ( 'NONE', *, *, #3428, .F. ) ;
#3528=PLANE ( 'NONE',  #7058 ) ;
#3533=EDGE_CURVE ( 'NONE', #5749, #4086, #1173, .T. ) ;
#3537=CIRCLE ( 'NONE', #5175, 5.999999999999991118 ) ;
#3544=FACE_OUTER_BOUND ( 'NONE', #2400, .T. ) ;
#3548=LINE ( 'NONE', #6127, #2908 ) ;
#3552=CARTESIAN_POINT ( 'NONE',  ( 0.000000000000000000, 0.000000000000000000, 20.00000000000000355 ) ) ;
#3559=ORIENTED_EDGE ( 'NONE', *, *, #1866, .T. ) ;
#3561=DIRECTION ( 'NONE',  ( 1.000000000000000000, 0.000000000000000000, 0.000000000000000000 ) ) ;
#3565=VECTOR ( 'NONE', #2360, 1000.000000000000000 ) ;
#3566=FACE_OUTER_BOUND ( 'NONE', #478, .T. ) ;
#3567=ORIENTED_EDGE ( 'NONE', *, *, #3333, .F. ) ;
#3570=EDGE_LOOP ( 'NONE', ( #481, #2833, #1003 ) ) ;
#3573=DIRECTION ( 'NONE',  ( 1.000000000000000000, 0.000000000000000000, 0.000000000000000000 ) ) ;
#3578=AXIS2_PLACEMENT_3D ( 'NONE', #4517, #3256, #5167 ) ;
#3595=VERTEX_POINT ( 'NONE', #3211 ) ;
#3618=AXIS2_PLACEMENT_3D ( 'NONE', #3496, #1074, #6850 ) ;
#3655=FACE_BOUND ( 'NONE', #7621, .T. ) ;
#3656=VERTEX_POINT ( 'NONE', #3935 ) ;
#3659=ORIENTED_EDGE ( 'NONE', *, *, #4069, .T. ) ;
#3661=EDGE_LOOP ( 'NONE', ( #2344, #845, #3681, #2107 ) ) ;
#3665=AXIS2_PLACEMENT_3D ( 'NONE', #1526, #4643, #3438 ) ;
#3675=DIRECTION ( 'NONE',  ( -1.000000000000000000, 0.000000000000000000, 0.000000000000000000 ) ) ;
#3681=ORIENTED_EDGE ( 'NONE', *, *, #8009, .T. ) ;
#3682=DIRECTION ( 'NONE',  ( 1.000000000000000000, 0.000000000000000000, 0.000000000000000000 ) ) ;
#3685=DIRECTION ( 'NONE',  ( -0.000000000000000000, -0.000000000000000000, 1.000000000000000000 ) ) ;
#3688=CARTESIAN_POINT ( 'NONE',  ( -115.0000000000000284, -115.0000000000000000, 20.00000000000000355 ) ) ;
#3697=UNCERTAINTY_MEASURE_WITH_UNIT (LENGTH_MEASURE( 1.000000000000000082E-05 ), #6897, 'distance_accuracy_value', 'NONE');
#3707=ADVANCED_FACE ( 'NONE', ( #5993 ), #6823, .F. ) ;
#3725=VERTEX_POINT ( 'NONE', #6716 ) ;
#3728=ORIENTED_EDGE ( 'NONE', *, *, #226, .F. ) ;
#3732=DIRECTION ( 'NONE',  ( -0.000000000000000000, -0.000000000000000000, -1.000000000000000000 ) ) ;
#3750=CARTESIAN_POINT ( 'NONE',  ( -109.0000000000000142, 115.0000000000000000, 20.00000000000000355 ) ) ;
#3762=PLANE ( 'NONE',  #2951 ) ;
#3763=EDGE_CURVE ( 'NONE', #1277, #8341, #4664, .T. ) ;
#3779=AXIS2_PLACEMENT_3D ( 'NONE', #6581, #7903, #7260 ) ;
#3780=ORIENTED_EDGE ( 'NONE', *, *, #3807, .T. ) ;
#3791=ORIENTED_EDGE ( 'NONE', *, *, #7652, .F. ) ;
#3795=DIRECTION ( 'NONE',  ( -1.000000000000000000, 0.000000000000000000, 0.000000000000000000 ) ) ;
#3807=EDGE_CURVE ( 'NONE', #8152, #4172, #5745, .T. ) ;
#3809=EDGE_CURVE ( 'NONE', #6480, #5338, #1583, .T. ) ;
#3811=CIRCLE ( 'NONE', #3665, 95.00000000000008527 ) ;
#3821=DIRECTION ( 'NONE',  ( 1.460819769243626145E-16, -1.000000000000000000, 0.000000000000000000 ) ) ;
#3823=LINE ( 'NONE', #7034, #6819 ) ;
#3824=DIRECTION ( 'NONE',  ( -0.000000000000000000, -0.000000000000000000, -1.000000000000000000 ) ) ;
#3832=DIRECTION ( 'NONE',  ( -0.000000000000000000, -0.000000000000000000, -1.000000000000000000 ) ) ;
#3834=ORIENTED_EDGE ( 'NONE', *, *, #3809, .F. ) ;
#3838=FACE_OUTER_BOUND ( 'NONE', #588, .T. ) ;
#3853=PLANE ( 'NONE',  #2266 ) ;
#3855=CIRCLE ( 'NONE', #5473, 5.999999999999991118 ) ;
#3859=ADVANCED_FACE ( 'NONE', ( #1979 ), #3853, .F. ) ;
#3869=CYLINDRICAL_SURFACE ( 'NONE', #7339, 5.999999999999991118 ) ;
#3871=CARTESIAN_POINT ( 'NONE',  ( 0.000000000000000000, 0.000000000000000000, 35.00000000000000000 ) ) ;
#3878=LINE ( 'NONE', #2093, #738 ) ;
#3883=ADVANCED_FACE ( 'NONE', ( #5068 ), #3182, .F. ) ;
#3893=CARTESIAN_POINT ( 'NONE',  ( 95.00000000000002842, -95.00000000000002842, 35.00000000000000000 ) ) ;
#3910=EDGE_CURVE ( 'NONE', #5894, #4086, #4278, .T. ) ;
#3922=DIRECTION ( 'NONE',  ( 0.000000000000000000, 1.000000000000000000, 0.000000000000000000 ) ) ;
#3935=CARTESIAN_POINT ( 'NONE',  ( -75.00000000000001421, 0.000000000000000000, 20.00000000000000355 ) ) ;
#3938=ORIENTED_EDGE ( 'NONE', *, *, #7686, .T. ) ;
#3955=DIRECTION ( 'NONE',  ( -0.000000000000000000, -0.000000000000000000, 1.000000000000000000 ) ) ;
#3967=LINE ( 'NONE', #6545, #3452 ) ;
#3968=DIRECTION ( 'NONE',  ( 0.000000000000000000, -1.000000000000000000, 0.000000000000000000 ) ) ;
#3974=ORIENTED_EDGE ( 'NONE', *, *, #4192, .F. ) ;
#3990=ORIENTED_EDGE ( 'NONE', *, *, #226, .T. ) ;
#3991=EDGE_CURVE ( 'NONE', #4671, #7451, #7586, .T. ) ;
#3999=VECTOR ( 'NONE', #1194, 1000.000000000000000 ) ;
#4002=CARTESIAN_POINT ( 'NONE',  ( 109.0000000000000142, 115.0000000000000000, 20.00000000000000355 ) ) ;
#4009=DIRECTION ( 'NONE',  ( -0.000000000000000000, -0.000000000000000000, 1.000000000000000000 ) ) ;
#4020=VECTOR ( 'NONE', #3685, 1000.000000000000000 ) ;
#4033=ORIENTED_EDGE ( 'NONE', *, *, #3910, .T. ) ;
#4055=CYLINDRICAL_SURFACE ( 'NONE', #390, 5.999999999999991118 ) ;
#4056=CARTESIAN_POINT ( 'NONE',  ( 0.000000000000000000, 0.000000000000000000, 0.000000000000000000 ) ) ;
#4063=DIRECTION ( 'NONE',  ( -0.000000000000000000, -0.000000000000000000, -1.000000000000000000 ) ) ;
#4069=EDGE_CURVE ( 'NONE', #7451, #984, #3548, .T. ) ;
#4081=PLANE ( 'NONE',  #5370 ) ;
#4086=VERTEX_POINT ( 'NONE', #3049 ) ;
#4092=EDGE_CURVE ( 'NONE', #7828, #431, #4999, .T. ) ;
#4097=ORIENTED_EDGE ( 'NONE', *, *, #1484, .F. ) ;
#4099=ADVANCED_FACE ( 'NONE', ( #6309 ), #2530, .F. ) ;
#4144=ORIENTED_EDGE ( 'NONE', *, *, #3375, .T. ) ;
#4156=EDGE_LOOP ( 'NONE', ( #3081, #4415, #4356 ) ) ;
#4159=CARTESIAN_POINT ( 'NONE',  ( 114.9999999999999858, 115.0000000000000000, 16.39483628583463570 ) ) ;
#4169=EDGE_LOOP ( 'NONE', ( #5143, #3938, #5437, #899, #1684 ) ) ;
#4172=VERTEX_POINT ( 'NONE', #5078 ) ;
#4173=LINE ( 'NONE', #8114, #4677 ) ;
#4179=CARTESIAN_POINT ( 'NONE',  ( 125.0000000000000000, 125.0000000000000284, 70.00000000000000000 ) ) ;
#4187=DIRECTION ( 'NONE',  ( -0.000000000000000000, -0.000000000000000000, -1.000000000000000000 ) ) ;
#4188=AXIS2_PLACEMENT_3D ( 'NONE', #5402, #7979, #7266 ) ;
#4192=EDGE_CURVE ( 'NONE', #5586, #3125, #3216, .T. ) ;
#4198=PRODUCT_DEFINITION_FORMATION_WITH_SPECIFIED_SOURCE ( 'ANY', '', #5128, .NOT_KNOWN. ) ;
#4199=CARTESIAN_POINT ( 'NONE',  ( 125.0000000000000000, 125.0000000000000284, 0.000000000000000000 ) ) ;
#4218=DIRECTION ( 'NONE',  ( 1.000000000000000000, 0.000000000000000000, 0.000000000000000000 ) ) ;
#4221=EDGE_LOOP ( 'NONE', ( #1396, #1096, #4705, #4279, #4585 ) ) ;
#4232=EDGE_LOOP ( 'NONE', ( #4915, #5130, #8227, #169, #1852 ) ) ;
#4236=VECTOR ( 'NONE', #2754, 1000.000000000000000 ) ;
#4260=VECTOR ( 'NONE', #5978, 1000.000000000000000 ) ;
#4269=ORIENTED_EDGE ( 'NONE', *, *, #2815, .F. ) ;
#4275=EDGE_LOOP ( 'NONE', ( #7611, #2689, #6241 ) ) ;
#4278=LINE ( 'NONE', #3750, #2659 ) ;
#4279=ORIENTED_EDGE ( 'NONE', *, *, #5716, .F. ) ;
#4290=ORIENTED_EDGE ( 'NONE', *, *, #7429, .T. ) ;
#4301=CARTESIAN_POINT ( 'NONE',  ( -115.0000000000000000, 115.0000000000000000, 20.00000000000000355 ) ) ;
#4305=LINE ( 'NONE', #2015, #5109 ) ;
#4314=VERTEX_POINT ( 'NONE', #1455 ) ;
#4318=DIRECTION ( 'NONE',  ( -0.000000000000000000, -0.000000000000000000, 1.000000000000000000 ) ) ;
#4326=CARTESIAN_POINT ( 'NONE',  ( 109.0000000000000426, -115.0000000000000000, 70.00000000000000000 ) ) ;
#4328=CIRCLE ( 'NONE', #4188, 5.999999999999991118 ) ;
#4335=ORIENTED_EDGE ( 'NONE', *, *, #8225, .T. ) ;
#4342=ORIENTED_EDGE ( 'NONE', *, *, #6688, .T. ) ;
#4351=CARTESIAN_POINT ( 'NONE',  ( 95.00000000000002842, -95.00000000000002842, 35.00000000000000000 ) ) ;
#4356=ORIENTED_EDGE ( 'NONE', *, *, #3533, .T. ) ;
#4360=ORIENTED_EDGE ( 'NONE', *, *, #2632, .T. ) ;
#4365=EDGE_LOOP ( 'NONE', ( #4926, #6002, #6830, #1773 ) ) ;
#4369=ORIENTED_EDGE ( 'NONE', *, *, #6489, .F. ) ;
#4371=DIRECTION ( 'NONE',  ( 1.000000000000000000, 0.000000000000000000, 0.000000000000000000 ) ) ;
#4372=ADVANCED_FACE ( 'NONE', ( #2793, #5298 ), #7880, .T. ) ;
#4375=VERTEX_POINT ( 'NONE', #7317 ) ;
#4384=VECTOR ( 'NONE', #2402, 1000.000000000000000 ) ;
#4395=ORIENTED_EDGE ( 'NONE', *, *, #1188, .T. ) ;
#4399=DIRECTION ( 'NONE',  ( -0.000000000000000000, -0.000000000000000000, 1.000000000000000000 ) ) ;
#4406=SHAPE_DEFINITION_REPRESENTATION ( #2064, #2264 ) ;
#4411=EDGE_LOOP ( 'NONE', ( #3728, #6727, #8018, #1452, #3032 ) ) ;
#4412=AXIS2_PLACEMENT_3D ( 'NONE', #1668, #7417, #6086 ) ;
#4413=VERTEX_POINT ( 'NONE', #6294 ) ;
#4415=ORIENTED_EDGE ( 'NONE', *, *, #3089, .T. ) ;
#4422=CIRCLE ( 'NONE', #4982, 5.999999999999991118 ) ;
#4430=EDGE_LOOP ( 'NONE', ( #4097, #6291, #2611, #357 ) ) ;
#4431=EDGE_CURVE ( 'NONE', #984, #431, #4173, .T. ) ;
#4441=CARTESIAN_POINT ( 'NONE',  ( 121.0000000000000000, 115.0000000000000000, 20.00000000000000355 ) ) ;
#4444=VERTEX_POINT ( 'NONE', #1071 ) ;
#4448=CARTESIAN_POINT ( 'NONE',  ( 121.0000000000000284, -115.0000000000000000, 70.00000000000000000 ) ) ;
#4456=DIRECTION ( 'NONE',  ( -0.000000000000000000, -0.000000000000000000, 1.000000000000000000 ) ) ;
#4465=DIRECTION ( 'NONE',  ( 0.000000000000000000, 0.000000000000000000, -1.000000000000000000 ) ) ;
#4517=CARTESIAN_POINT ( 'NONE',  ( 115.0000000000000000, 115.0000000000000000, 20.00000000000000355 ) ) ;
#4530=LINE ( 'NONE', #4707, #5913 ) ;
#4539=AXIS2_PLACEMENT_3D ( 'NONE', #5214, #2687, #5266 ) ;
#4556=VECTOR ( 'NONE', #999, 1000.000000000000000 ) ;
#4562=ORIENTED_EDGE ( 'NONE', *, *, #8095, .T. ) ;
#4575=CARTESIAN_POINT ( 'NONE',  ( -75.00000000000001421, 0.000000000000000000, 35.00000000000000000 ) ) ;
#4585=ORIENTED_EDGE ( 'NONE', *, *, #6489, .T. ) ;
#4589=CARTESIAN_POINT ( 'NONE',  ( -109.0000000000000426, -115.0000000000000000, 70.00000000000000000 ) ) ;
#4595=DIRECTION ( 'NONE',  ( 1.460819769243625652E-16, -1.000000000000000000, -0.000000000000000000 ) ) ;
#4599=LINE ( 'NONE', #6542, #2516 ) ;
#4609=CIRCLE ( 'NONE', #2085, 95.00000000000008527 ) ;
#4614=( NAMED_UNIT ( * ) SI_UNIT ( $, .STERADIAN. ) SOLID_ANGLE_UNIT ( ) );
#4615=AXIS2_PLACEMENT_3D ( 'NONE', #8081, #394, #2313 ) ;
#4637=ORIENTED_EDGE ( 'NONE', *, *, #8257, .F. ) ;
#4643=DIRECTION ( 'NONE',  ( 0.000000000000000000, 0.000000000000000000, 1.000000000000000000 ) ) ;
#4645=DIRECTION ( 'NONE',  ( -1.000000000000000000, 0.000000000000000000, -0.000000000000000000 ) ) ;
#4648=VERTEX_POINT ( 'NONE', #7711 ) ;
#4664=CIRCLE ( 'NONE', #7239, 5.999999999999991118 ) ;
#4665=DIRECTION ( 'NONE',  ( 1.000000000000000000, 0.000000000000000000, 0.000000000000000000 ) ) ;
#4671=VERTEX_POINT ( 'NONE', #3285 ) ;
#4677=VECTOR ( 'NONE', #5501, 1000.000000000000000 ) ;
#4693=CIRCLE ( 'NONE', #8062, 5.999999999999991118 ) ;
#4705=ORIENTED_EDGE ( 'NONE', *, *, #3991, .T. ) ;
#4706=DIRECTION ( 'NONE',  ( -0.000000000000000000, -0.000000000000000000, 1.000000000000000000 ) ) ;
#4707=CARTESIAN_POINT ( 'NONE',  ( -95.00000000000000000, 95.00000000000008527, 70.00000000000000000 ) ) ;
#4730=DIRECTION ( 'NONE',  ( 1.000000000000000000, 0.000000000000000000, 0.000000000000000000 ) ) ;
#4733=EDGE_CURVE ( 'NONE', #6616, #6102, #2221, .T. ) ;
#4739=CARTESIAN_POINT ( 'NONE',  ( 125.0000000000000000, -125.0000000000000284, 0.000000000000000000 ) ) ;
#4741=CARTESIAN_POINT ( 'NONE',  ( -94.99999999999997158, -95.00000000000008527, 35.00000000000000000 ) ) ;
#4745=EDGE_LOOP ( 'NONE', ( #2439, #4637, #1949, #6523 ) ) ;
#4766=LINE ( 'NONE', #3402, #4986 ) ;
#4776=EDGE_CURVE ( 'NONE', #7369, #5586, #1570, .T. ) ;
#4795=EDGE_CURVE ( 'NONE', #4444, #2571, #3967, .T. ) ;
#4800=DIRECTION ( 'NONE',  ( -1.000000000000000000, -1.460819769243626145E-16, 0.000000000000000000 ) ) ;
#4828=DIRECTION ( 'NONE',  ( -0.000000000000000000, -0.000000000000000000, 1.000000000000000000 ) ) ;
#4840=ORIENTED_EDGE ( 'NONE', *, *, #7172, .F. ) ;
#4845=VECTOR ( 'NONE', #1371, 1000.000000000000000 ) ;
#4846=EDGE_LOOP ( 'NONE', ( #3109, #2831, #8156 ) ) ;
#4852=CARTESIAN_POINT ( 'NONE',  ( 115.0000000000000000, 115.0000000000000000, 70.00000000000000000 ) ) ;
#4858=CARTESIAN_POINT ( 'NONE',  ( -115.0000000000000284, -115.0000000000000000, 20.00000000000000355 ) ) ;
#4871=LINE ( 'NONE', #2447, #3565 ) ;
#4876=DIRECTION ( 'NONE',  ( 1.000000000000000000, 0.000000000000000000, 0.000000000000000000 ) ) ;
#4882=DIRECTION ( 'NONE',  ( 0.000000000000000000, 0.000000000000000000, -1.000000000000000000 ) ) ;
#4885=DIRECTION ( 'NONE',  ( 1.000000000000000000, 0.000000000000000000, 0.000000000000000000 ) ) ;
#4890=DIRECTION ( 'NONE',  ( -0.000000000000000000, -0.000000000000000000, 1.000000000000000000 ) ) ;
#4914=FACE_OUTER_BOUND ( 'NONE', #2589, .T. ) ;
#4915=ORIENTED_EDGE ( 'NONE', *, *, #5965, .F. ) ;
#4918=DIRECTION ( 'NONE',  ( -0.000000000000000000, -0.000000000000000000, 1.000000000000000000 ) ) ;
#4926=ORIENTED_EDGE ( 'NONE', *, *, #8105, .T. ) ;
#4927=ADVANCED_FACE ( 'NONE', ( #3566 ), #1785, .F. ) ;
#4935=ORIENTED_EDGE ( 'NONE', *, *, #5829, .T. ) ;
#4957=DIRECTION ( 'NONE',  ( -0.000000000000000000, -0.000000000000000000, 1.000000000000000000 ) ) ;
#4958=EDGE_LOOP ( 'NONE', ( #3791, #567, #1310, #1577 ) ) ;
#4968=DIRECTION ( 'NONE',  ( 0.8571673007021112234, 0.000000000000000000, 0.5150380749100560429 ) ) ;
#4982=AXIS2_PLACEMENT_3D ( 'NONE', #4852, #2340, #6932 ) ;
#4986=VECTOR ( 'NONE', #1142, 1000.000000000000000 ) ;
#4997=EDGE_CURVE ( 'NONE', #7082, #5603, #682, .T. ) ;
#4999=LINE ( 'NONE', #1802, #7109 ) ;
#5001=AXIS2_PLACEMENT_3D ( 'NONE', #2986, #4890, #3488 ) ;
#5014=LINE ( 'NONE', #4326, #8102 ) ;
#5028=EDGE_CURVE ( 'NONE', #6392, #4671, #868, .T. ) ;
#5046=VECTOR ( 'NONE', #2566, 1000.000000000000000 ) ;
#5053=LINE ( 'NONE', #7644, #1766 ) ;
#5060=EDGE_CURVE ( 'NONE', #4375, #7541, #7655, .T. ) ;
#5068=FACE_OUTER_BOUND ( 'NONE', #5236, .T. ) ;
#5069=EDGE_LOOP ( 'NONE', ( #7950, #5092, #1994 ) ) ;
#5076=ORIENTED_EDGE ( 'NONE', *, *, #840, .F. ) ;
#5077=AXIS2_PLACEMENT_3D ( 'NONE', #7705, #4465, #3084 ) ;
#5078=CARTESIAN_POINT ( 'NONE',  ( -121.0000000000000284, -115.0000000000000000, 20.00000000000000355 ) ) ;
#5082=DIRECTION ( 'NONE',  ( -0.000000000000000000, -0.000000000000000000, 1.000000000000000000 ) ) ;
#5092=ORIENTED_EDGE ( 'NONE', *, *, #4795, .T. ) ;
#5093=CYLINDRICAL_SURFACE ( 'NONE', #7401, 75.00000000000001421 ) ;
#5106=APPLICATION_CONTEXT ( 'automotive_design' ) ;
#5109=VECTOR ( 'NONE', #7144, 1000.000000000000000 ) ;
#5118=EDGE_LOOP ( 'NONE', ( #2928, #6363, #887, #4562 ) ) ;
#5121=AXIS2_PLACEMENT_3D ( 'NONE', #7560, #2459, #251 ) ;
#5128=PRODUCT ( 'Bearing Housing', 'Bearing Housing', '', ( #2499 ) ) ;
#5130=ORIENTED_EDGE ( 'NONE', *, *, #1188, .F. ) ;
#5139=CARTESIAN_POINT ( 'NONE',  ( 115.0000000000000284, -115.0000000000000000, 70.00000000000000000 ) ) ;
#5143=ORIENTED_EDGE ( 'NONE', *, *, #4092, .T. ) ;
#5145=CARTESIAN_POINT ( 'NONE',  ( 125.0000000000000000, -125.0000000000000284, 0.000000000000000000 ) ) ;
#5167=DIRECTION ( 'NONE',  ( 1.000000000000000000, 0.000000000000000000, 0.000000000000000000 ) ) ;
#5175=AXIS2_PLACEMENT_3D ( 'NONE', #7557, #4318, #6920 ) ;
#5202=ORIENTED_EDGE ( 'NONE', *, *, #8009, .F. ) ;
#5213=DIRECTION ( 'NONE',  ( -0.000000000000000000, -0.000000000000000000, -1.000000000000000000 ) ) ;
#5214=CARTESIAN_POINT ( 'NONE',  ( -115.0000000000000284, -115.0000000000000000, 70.00000000000000000 ) ) ;
#5225=AXIS2_PLACEMENT_3D ( 'NONE', #1293, #6429, #5886 ) ;
#5236=EDGE_LOOP ( 'NONE', ( #1287, #3780, #5743 ) ) ;
#5262=DIRECTION ( 'NONE',  ( -1.000000000000000000, 0.000000000000000000, 0.000000000000000000 ) ) ;
#5266=DIRECTION ( 'NONE',  ( 1.000000000000000000, 0.000000000000000000, 0.000000000000000000 ) ) ;
#5288=DIRECTION ( 'NONE',  ( -0.000000000000000000, -1.000000000000000000, -0.000000000000000000 ) ) ;
#5298=FACE_BOUND ( 'NONE', #7852, .T. ) ;
#5303=LINE ( 'NONE', #4575, #7801 ) ;
#5317=EDGE_LOOP ( 'NONE', ( #7079, #2592, #4144, #96 ) ) ;
#5338=VERTEX_POINT ( 'NONE', #6061 ) ;
#5339=FACE_OUTER_BOUND ( 'NONE', #7399, .T. ) ;
#5365=CYLINDRICAL_SURFACE ( 'NONE', #5121, 5.999999999999991118 ) ;
#5370=AXIS2_PLACEMENT_3D ( 'NONE', #6674, #3968, #894 ) ;
#5372=ORIENTED_EDGE ( 'NONE', *, *, #8257, .T. ) ;
#5374=CIRCLE ( 'NONE', #6447, 95.00000000000008527 ) ;
#5385=CARTESIAN_POINT ( 'NONE',  ( -115.0000000000000000, 115.0000000000000000, 20.00000000000000355 ) ) ;
#5402=CARTESIAN_POINT ( 'NONE',  ( -115.0000000000000284, -115.0000000000000000, 20.00000000000000355 ) ) ;
#5407=CONICAL_SURFACE ( 'NONE', #5001, 5.999999999999991118, 1.029744258676652313 ) ;
#5425=CARTESIAN_POINT ( 'NONE',  ( 115.0000000000000000, 115.0000000000000000, 20.00000000000000355 ) ) ;
#5428=CARTESIAN_POINT ( 'NONE',  ( 2.775557561562893875E-14, -95.00000000000008527, 35.00000000000000000 ) ) ;
#5437=ORIENTED_EDGE ( 'NONE', *, *, #7172, .T. ) ;
#5439=VERTEX_POINT ( 'NONE', #1561 ) ;
#5452=ORIENTED_EDGE ( 'NONE', *, *, #6012, .T. ) ;
#5473=AXIS2_PLACEMENT_3D ( 'NONE', #5684, #5082, #7765 ) ;
#5476=DIRECTION ( 'NONE',  ( -0.000000000000000000, -0.000000000000000000, 1.000000000000000000 ) ) ;
#5478=ORIENTED_EDGE ( 'NONE', *, *, #6603, .F. ) ;
#5482=AXIS2_PLACEMENT_3D ( 'NONE', #3688, #4957, #2318 ) ;
#5501=DIRECTION ( 'NONE',  ( 1.000000000000000000, 0.000000000000000000, 0.000000000000000000 ) ) ;
#5506=ORIENTED_EDGE ( 'NONE', *, *, #1015, .F. ) ;
#5511=CIRCLE ( 'NONE', #2937, 5.999999999999991118 ) ;
#5512=PLANE ( 'NONE',  #4615 ) ;
#5517=ORIENTED_EDGE ( 'NONE', *, *, #1245, .F. ) ;
#5519=CARTESIAN_POINT ( 'NONE',  ( 95.00000000000008527, 0.000000000000000000, 20.00000000000000355 ) ) ;
#5529=ORIENTED_EDGE ( 'NONE', *, *, #5028, .F. ) ;
#5549=VECTOR ( 'NONE', #3955, 1000.000000000000000 ) ;
#5561=CARTESIAN_POINT ( 'NONE',  ( 95.00000000000002842, -95.00000000000002842, 70.00000000000000000 ) ) ;
#5575=EDGE_CURVE ( 'NONE', #4086, #5749, #5511, .T. ) ;
#5586=VERTEX_POINT ( 'NONE', #7685 ) ;
#5591=ORIENTED_EDGE ( 'NONE', *, *, #6012, .F. ) ;
#5602=CARTESIAN_POINT ( 'NONE',  ( 0.000000000000000000, 0.000000000000000000, 35.00000000000000000 ) ) ;
#5603=VERTEX_POINT ( 'NONE', #4448 ) ;
#5613=EDGE_LOOP ( 'NONE', ( #6810, #3659, #7090, #3492, #2052 ) ) ;
#5624=CARTESIAN_POINT ( 'NONE',  ( -121.0000000000000000, 115.0000000000000000, 20.00000000000000355 ) ) ;
#5664=DIRECTION ( 'NONE',  ( -0.000000000000000000, -0.000000000000000000, 1.000000000000000000 ) ) ;
#5668=ADVANCED_FACE ( 'NONE', ( #749 ), #7245, .F. ) ;
#5684=CARTESIAN_POINT ( 'NONE',  ( 115.0000000000000000, 115.0000000000000000, 20.00000000000000355 ) ) ;
#5692=FACE_BOUND ( 'NONE', #5861, .T. ) ;
#5709=PLANE ( 'NONE',  #858 ) ;
#5716=EDGE_CURVE ( 'NONE', #2612, #7451, #4530, .T. ) ;
#5727=AXIS2_PLACEMENT_3D ( 'NONE', #3426, #228, #7337 ) ;
#5735=FACE_OUTER_BOUND ( 'NONE', #1478, .T. ) ;
#5743=ORIENTED_EDGE ( 'NONE', *, *, #1197, .T. ) ;
#5745=LINE ( 'NONE', #3204, #215 ) ;
#5747=AXIS2_PLACEMENT_3D ( 'NONE', #1940, #1290, #11 ) ;
#5749=VERTEX_POINT ( 'NONE', #7773 ) ;
#5753=AXIS2_PLACEMENT_3D ( 'NONE', #4301, #389, #6766 ) ;
#5762=ADVANCED_FACE ( 'NONE', ( #7815 ), #311, .T. ) ;
#5778=DIRECTION ( 'NONE',  ( 1.000000000000000000, 0.000000000000000000, 0.000000000000000000 ) ) ;
#5781=CARTESIAN_POINT ( 'NONE',  ( -115.0000000000000426, -115.0000000000000000, 16.39483628583463570 ) ) ;
#5787=CIRCLE ( 'NONE', #6175, 95.00000000000008527 ) ;
#5788=CARTESIAN_POINT ( 'NONE',  ( 95.00000000000002842, -95.00000000000002842, 70.00000000000000000 ) ) ;
#5795=EDGE_CURVE ( 'NONE', #5876, #4314, #5787, .T. ) ;
#5804=AXIS2_PLACEMENT_3D ( 'NONE', #5139, #2497, #3233 ) ;
#5810=DIRECTION ( 'NONE',  ( -0.000000000000000000, -0.000000000000000000, -1.000000000000000000 ) ) ;
#5817=CARTESIAN_POINT ( 'NONE',  ( 0.000000000000000000, 0.000000000000000000, 35.00000000000000000 ) ) ;
#5827=DIRECTION ( 'NONE',  ( 0.000000000000000000, 0.000000000000000000, 1.000000000000000000 ) ) ;
#5829=EDGE_CURVE ( 'NONE', #3069, #5876, #1085, .T. ) ;
#5831=CIRCLE ( 'NONE', #2849, 5.999999999999991118 ) ;
#5861=EDGE_LOOP ( 'NONE', ( #1414, #7746 ) ) ;
#5876=VERTEX_POINT ( 'NONE', #5428 ) ;
#5880=STYLED_ITEM('',(#8400),#3512);
#5884=CARTESIAN_POINT ( 'NONE',  ( 0.000000000000000000, 0.000000000000000000, 0.000000000000000000 ) ) ;
#5886=DIRECTION ( 'NONE',  ( 1.000000000000000000, 0.000000000000000000, 0.000000000000000000 ) ) ;
#5894=VERTEX_POINT ( 'NONE', #2802 ) ;
#5897=VECTOR ( 'NONE', #5288, 1000.000000000000000 ) ;
#5902=CARTESIAN_POINT ( 'NONE',  ( -121.0000000000000000, 115.0000000000000000, 70.00000000000000000 ) ) ;
#5912=AXIS2_PLACEMENT_3D ( 'NONE', #3552, #7461, #6131 ) ;
#5913=VECTOR ( 'NONE', #4063, 1000.000000000000000 ) ;
#5919=CARTESIAN_POINT ( 'NONE',  ( -115.0000000000000284, -115.0000000000000000, 70.00000000000000000 ) ) ;
#5927=DIRECTION ( 'NONE',  ( 1.000000000000000000, 0.000000000000000000, 0.000000000000000000 ) ) ;
#5935=DIRECTION ( 'NONE',  ( -1.000000000000000000, 0.000000000000000000, -0.000000000000000000 ) ) ;
#5937=VERTEX_POINT ( 'NONE', #2671 ) ;
#5943=AXIS2_PLACEMENT_3D ( 'NONE', #8019, #4800, #2295 ) ;
#5948=AXIS2_PLACEMENT_3D ( 'NONE', #318, #5476, #2885 ) ;
#5965=EDGE_CURVE ( 'NONE', #3065, #4671, #80, .T. ) ;
#5966=CARTESIAN_POINT ( 'NONE',  ( 115.0000000000000000, 115.0000000000000000, 70.00000000000000000 ) ) ;
#5967=( LENGTH_UNIT ( ) NAMED_UNIT ( * ) SI_UNIT ( .MILLI., .METRE. ) );
#5978=DIRECTION ( 'NONE',  ( -0.000000000000000000, -0.000000000000000000, -1.000000000000000000 ) ) ;
#5985=CARTESIAN_POINT ( 'NONE',  ( 75.00000000000001421, 9.184850993605150311E-15, 0.000000000000000000 ) ) ;
#5993=FACE_OUTER_BOUND ( 'NONE', #5069, .T. ) ;
#5995=ORIENTED_EDGE ( 'NONE', *, *, #7896, .F. ) ;
#6002=ORIENTED_EDGE ( 'NONE', *, *, #4776, .T. ) ;
#6009=CARTESIAN_POINT ( 'NONE',  ( -125.0000000000000000, -125.0000000000000284, 0.000000000000000000 ) ) ;
#6012=EDGE_CURVE ( 'NONE', #7934, #7988, #4305, .T. ) ;
#6014=VECTOR ( 'NONE', #6812, 1000.000000000000000 ) ;
#6061=CARTESIAN_POINT ( 'NONE',  ( -75.00000000000001421, 0.000000000000000000, 0.000000000000000000 ) ) ;
#6078=DIRECTION ( 'NONE',  ( 1.000000000000000000, 0.000000000000000000, 0.000000000000000000 ) ) ;
#6086=DIRECTION ( 'NONE',  ( -1.460819769243625652E-16, 1.000000000000000000, 0.000000000000000000 ) ) ;
#6102=VERTEX_POINT ( 'NONE', #6595 ) ;
#6125=FACE_BOUND ( 'NONE', #7445, .T. ) ;
#6127=CARTESIAN_POINT ( 'NONE',  ( 95.00000000000000000, 95.00000000000008527, 35.00000000000000000 ) ) ;
#6131=DIRECTION ( 'NONE',  ( 1.000000000000000000, 0.000000000000000000, 0.000000000000000000 ) ) ;
#6133=AXIS2_PLACEMENT_3D ( 'NONE', #23, #590, #7777 ) ;
#6135=FACE_OUTER_BOUND ( 'NONE', #4411, .T. ) ;
#6136=VECTOR ( 'NONE', #6563, 1000.000000000000000 ) ;
#6165=VECTOR ( 'NONE', #635, 1000.000000000000000 ) ;
#6175=AXIS2_PLACEMENT_3D ( 'NONE', #2243, #398, #4218 ) ;
#6183=FACE_OUTER_BOUND ( 'NONE', #7358, .T. ) ;
#6199=PLANE ( 'NONE',  #5943 ) ;
#6221=EDGE_LOOP ( 'NONE', ( #2165, #5517 ) ) ;
#6241=ORIENTED_EDGE ( 'NONE', *, *, #4069, .F. ) ;
#6278=EDGE_CURVE ( 'NONE', #8341, #1277, #4422, .T. ) ;
#6291=ORIENTED_EDGE ( 'NONE', *, *, #3333, .T. ) ;
#6294=CARTESIAN_POINT ( 'NONE',  ( -125.0000000000000000, 125.0000000000000284, 0.000000000000000000 ) ) ;
#6309=FACE_OUTER_BOUND ( 'NONE', #3570, .T. ) ;
#6343=ADVANCED_FACE ( 'NONE', ( #7136 ), #3762, .F. ) ;
#6351=AXIS2_PLACEMENT_3D ( 'NONE', #6695, #4187, #4876 ) ;
#6362=DIRECTION ( 'NONE',  ( 0.000000000000000000, -0.000000000000000000, -1.000000000000000000 ) ) ;
#6363=ORIENTED_EDGE ( 'NONE', *, *, #530, .F. ) ;
#6365=ORIENTED_EDGE ( 'NONE', *, *, #6278, .F. ) ;
#6366=CIRCLE ( 'NONE', #148, 5.999999999999991118 ) ;
#6367=CARTESIAN_POINT ( 'NONE',  ( 125.0000000000000000, -125.0000000000000284, 70.00000000000000000 ) ) ;
#6375=FACE_OUTER_BOUND ( 'NONE', #1783, .T. ) ;
#6379=CARTESIAN_POINT ( 'NONE',  ( 95.00000000000002842, -95.00000000000002842, 35.00000000000000000 ) ) ;
#6392=VERTEX_POINT ( 'NONE', #555 ) ;
#6395=ORIENTED_EDGE ( 'NONE', *, *, #1245, .T. ) ;
#6415=ORIENTED_EDGE ( 'NONE', *, *, #1866, .F. ) ;
#6429=DIRECTION ( 'NONE',  ( -0.000000000000000000, -0.000000000000000000, 1.000000000000000000 ) ) ;
#6440=CARTESIAN_POINT ( 'NONE',  ( 95.00000000000002842, -95.00000000000002842, 35.00000000000000000 ) ) ;
#6441=CARTESIAN_POINT ( 'NONE',  ( 125.0000000000000000, 125.0000000000000284, 70.00000000000000000 ) ) ;
#6444=AXIS2_PLACEMENT_3D ( 'NONE', #985, #8069, #3573 ) ;
#6447=AXIS2_PLACEMENT_3D ( 'NONE', #5817, #20, #7775 ) ;
#6454=ORIENTED_EDGE ( 'NONE', *, *, #419, .T. ) ;
#6473=CARTESIAN_POINT ( 'NONE',  ( 109.0000000000000142, 115.0000000000000000, 70.00000000000000000 ) ) ;
#6477=VERTEX_POINT ( 'NONE', #5902 ) ;
#6480=VERTEX_POINT ( 'NONE', #5985 ) ;
#6489=EDGE_CURVE ( 'NONE', #2612, #7934, #194, .T. ) ;
#6494=VERTEX_POINT ( 'NONE', #761 ) ;
#6498=AXIS2_PLACEMENT_3D ( 'NONE', #3461, #4706, #1423 ) ;
#6500=DIRECTION ( 'NONE',  ( 0.000000000000000000, 1.000000000000000000, 0.000000000000000000 ) ) ;
#6513=ADVANCED_FACE ( 'NONE', ( #2816 ), #2212, .F. ) ;
#6518=DIRECTION ( 'NONE',  ( 0.000000000000000000, 0.000000000000000000, -1.000000000000000000 ) ) ;
#6523=ORIENTED_EDGE ( 'NONE', *, *, #2815, .T. ) ;
#6542=CARTESIAN_POINT ( 'NONE',  ( 125.0000000000000000, -125.0000000000000284, 0.000000000000000000 ) ) ;
#6545=CARTESIAN_POINT ( 'NONE',  ( 109.0000000000000426, -115.0000000000000000, 20.00000000000000355 ) ) ;
#6563=DIRECTION ( 'NONE',  ( 1.000000000000000000, -0.000000000000000000, -0.000000000000000000 ) ) ;
#6566=PLANE ( 'NONE',  #646 ) ;
#6581=CARTESIAN_POINT ( 'NONE',  ( -115.0000000000000000, 115.0000000000000000, 70.00000000000000000 ) ) ;
#6595=CARTESIAN_POINT ( 'NONE',  ( 109.0000000000000142, 115.0000000000000000, 20.00000000000000355 ) ) ;
#6603=EDGE_CURVE ( 'NONE', #7828, #2612, #6874, .T. ) ;
#6609=LINE ( 'NONE', #867, #6136 ) ;
#6612=DIRECTION ( 'NONE',  ( 1.000000000000000000, 0.000000000000000000, 0.000000000000000000 ) ) ;
#6616=VERTEX_POINT ( 'NONE', #4159 ) ;
#6636=ORIENTED_EDGE ( 'NONE', *, *, #1197, .F. ) ;
#6642=ADVANCED_FACE ( 'NONE', ( #410 ), #324, .F. ) ;
#6674=CARTESIAN_POINT ( 'NONE',  ( 95.00000000000000000, 95.00000000000008527, 70.00000000000000000 ) ) ;
#6687=CONICAL_SURFACE ( 'NONE', #7370, 5.999999999999991118, 1.029744258676652313 ) ;
#6688=EDGE_CURVE ( 'NONE', #8152, #3595, #2854, .T. ) ;
#6695=CARTESIAN_POINT ( 'NONE',  ( 0.000000000000000000, 0.000000000000000000, 20.00000000000000355 ) ) ;
#6696=VECTOR ( 'NONE', #7802, 1000.000000000000000 ) ;
#6698=ORIENTED_EDGE ( 'NONE', *, *, #4795, .F. ) ;
#6716=CARTESIAN_POINT ( 'NONE',  ( 121.0000000000000000, 115.0000000000000000, 20.00000000000000355 ) ) ;
#6727=ORIENTED_EDGE ( 'NONE', *, *, #5965, .T. ) ;
#6731=CARTESIAN_POINT ( 'NONE',  ( -109.0000000000000142, 115.0000000000000000, 70.00000000000000000 ) ) ;
#6742=DIRECTION ( 'NONE',  ( -0.000000000000000000, -0.000000000000000000, 1.000000000000000000 ) ) ;
#6760=ORIENTED_EDGE ( 'NONE', *, *, #31, .T. ) ;
#6766=DIRECTION ( 'NONE',  ( 1.000000000000000000, 0.000000000000000000, 0.000000000000000000 ) ) ;
#6779=PRODUCT_DEFINITION_CONTEXT ( 'detailed design', #8075, 'design' ) ;
#6804=ADVANCED_FACE ( 'NONE', ( #5735 ), #5093, .F. ) ;
#6810=ORIENTED_EDGE ( 'NONE', *, *, #5716, .T. ) ;
#6811=ADVANCED_FACE ( 'NONE', ( #1182 ), #519, .F. ) ;
#6812=DIRECTION ( 'NONE',  ( -1.460819769243625652E-16, 1.000000000000000000, 0.000000000000000000 ) ) ;
#6813=EDGE_CURVE ( 'NONE', #4314, #984, #5374, .T. ) ;
#6819=VECTOR ( 'NONE', #5213, 1000.000000000000000 ) ;
#6823=CONICAL_SURFACE ( 'NONE', #2774, 5.999999999999991118, 1.029744258676652313 ) ;
#6828=CARTESIAN_POINT ( 'NONE',  ( 95.00000000000002842, -95.00000000000002842, 70.00000000000000000 ) ) ;
#6830=ORIENTED_EDGE ( 'NONE', *, *, #3428, .T. ) ;
#6834=FACE_OUTER_BOUND ( 'NONE', #1286, .T. ) ;
#6850=DIRECTION ( 'NONE',  ( 1.000000000000000000, 0.000000000000000000, 0.000000000000000000 ) ) ;
#6857=VECTOR ( 'NONE', #7508, 1000.000000000000000 ) ;
#6863=CYLINDRICAL_SURFACE ( 'NONE', #5912, 95.00000000000008527 ) ;
#6867=CYLINDRICAL_SURFACE ( 'NONE', #5225, 5.999999999999991118 ) ;
#6874=LINE ( 'NONE', #8138, #6857 ) ;
#6897=( LENGTH_UNIT ( ) NAMED_UNIT ( * ) SI_UNIT ( .MILLI., .METRE. ) );
#6920=DIRECTION ( 'NONE',  ( 1.000000000000000000, 0.000000000000000000, 0.000000000000000000 ) ) ;
#6921=ORIENTED_EDGE ( 'NONE', *, *, #2388, .F. ) ;
#6932=DIRECTION ( 'NONE',  ( 1.000000000000000000, 0.000000000000000000, 0.000000000000000000 ) ) ;
#6938=DIRECTION ( 'NONE',  ( 0.000000000000000000, 0.000000000000000000, 1.000000000000000000 ) ) ;
#6946=CARTESIAN_POINT ( 'NONE',  ( -95.00000000000008527, 1.163414459189986590E-14, 20.00000000000000355 ) ) ;
#6973=ORIENTED_EDGE ( 'NONE', *, *, #8157, .T. ) ;
#6989=CARTESIAN_POINT ( 'NONE',  ( 75.00000000000001421, 9.184850993605150311E-15, 35.00000000000000000 ) ) ;
#7034=CARTESIAN_POINT ( 'NONE',  ( -125.0000000000000000, 125.0000000000000284, 70.00000000000000000 ) ) ;
#7050=DIRECTION ( 'NONE',  ( 0.000000000000000000, 1.000000000000000000, -0.000000000000000000 ) ) ;
#7058=AXIS2_PLACEMENT_3D ( 'NONE', #7983, #1528, #4645 ) ;
#7077=EDGE_CURVE ( 'NONE', #3725, #1277, #400, .T. ) ;
#7079=ORIENTED_EDGE ( 'NONE', *, *, #2474, .F. ) ;
#7082=VERTEX_POINT ( 'NONE', #269 ) ;
#7090=ORIENTED_EDGE ( 'NONE', *, *, #4431, .T. ) ;
#7109=VECTOR ( 'NONE', #3732, 1000.000000000000000 ) ;
#7114=ADVANCED_FACE ( 'NONE', ( #2317 ), #6863, .F. ) ;
#7128=DIRECTION ( 'NONE',  ( -0.8571673007021112234, 1.049727191138617340E-16, 0.5150380749100560429 ) ) ;
#7129=VECTOR ( 'NONE', #4595, 1000.000000000000000 ) ;
#7136=FACE_OUTER_BOUND ( 'NONE', #7721, .T. ) ;
#7141=ORIENTED_EDGE ( 'NONE', *, *, #3394, .F. ) ;
#7144=DIRECTION ( 'NONE',  ( 1.000000000000000000, 2.921639538487254261E-16, -0.000000000000000000 ) ) ;
#7171=LINE ( 'NONE', #4589, #5549 ) ;
#7172=EDGE_CURVE ( 'NONE', #4314, #3069, #3217, .T. ) ;
#7198=CARTESIAN_POINT ( 'NONE',  ( -125.0000000000000000, -125.0000000000000284, 0.000000000000000000 ) ) ;
#7226=CARTESIAN_POINT ( 'NONE',  ( 95.00000000000000000, 95.00000000000008527, 70.00000000000000000 ) ) ;
#7239=AXIS2_PLACEMENT_3D ( 'NONE', #363, #7476, #3561 ) ;
#7245=PLANE ( 'NONE',  #2553 ) ;
#7260=DIRECTION ( 'NONE',  ( 1.000000000000000000, 0.000000000000000000, 0.000000000000000000 ) ) ;
#7266=DIRECTION ( 'NONE',  ( 1.000000000000000000, 0.000000000000000000, 0.000000000000000000 ) ) ;
#7273=CARTESIAN_POINT ( 'NONE',  ( 125.0000000000000000, 125.0000000000000284, 70.00000000000000000 ) ) ;
#7279=CIRCLE ( 'NONE', #3618, 95.00000000000008527 ) ;
#7291=DIRECTION ( 'NONE',  ( -0.000000000000000000, -0.000000000000000000, 1.000000000000000000 ) ) ;
#7297=CARTESIAN_POINT ( 'NONE',  ( -94.99999999999997158, -95.00000000000008527, 70.00000000000000000 ) ) ;
#7307=FACE_OUTER_BOUND ( 'NONE', #5613, .T. ) ;
#7317=CARTESIAN_POINT ( 'NONE',  ( 125.0000000000000000, -125.0000000000000284, 70.00000000000000000 ) ) ;
#7331=ORIENTED_EDGE ( 'NONE', *, *, #4733, .T. ) ;
#7336=ADVANCED_FACE ( 'NONE', ( #2684 ), #4055, .F. ) ;
#7337=DIRECTION ( 'NONE',  ( 1.000000000000000000, 0.000000000000000000, 0.000000000000000000 ) ) ;
#7338=CYLINDRICAL_SURFACE ( 'NONE', #2593, 5.999999999999991118 ) ;
#7339=AXIS2_PLACEMENT_3D ( 'NONE', #3505, #313, #4665 ) ;
#7358=EDGE_LOOP ( 'NONE', ( #750, #4342, #2161 ) ) ;
#7360=CARTESIAN_POINT ( 'NONE',  ( 0.000000000000000000, 0.000000000000000000, 0.000000000000000000 ) ) ;
#7361=AXIS2_PLACEMENT_3D ( 'NONE', #6441, #675, #6362 ) ;
#7369=VERTEX_POINT ( 'NONE', #865 ) ;
#7370=AXIS2_PLACEMENT_3D ( 'NONE', #8177, #1090, #1002 ) ;
#7399=EDGE_LOOP ( 'NONE', ( #294, #4033, #492 ) ) ;
#7401=AXIS2_PLACEMENT_3D ( 'NONE', #3871, #3832, #8318 ) ;
#7405=ORIENTED_EDGE ( 'NONE', *, *, #396, .F. ) ;
#7417=DIRECTION ( 'NONE',  ( 1.000000000000000000, 1.460819769243625652E-16, -0.000000000000000000 ) ) ;
#7428=DIRECTION ( 'NONE',  ( -1.460819769243626145E-16, 1.000000000000000000, 0.000000000000000000 ) ) ;
#7429=EDGE_CURVE ( 'NONE', #5749, #6477, #784, .T. ) ;
#7440=DIRECTION ( 'NONE',  ( -0.000000000000000000, -0.000000000000000000, 1.000000000000000000 ) ) ;
#7445=EDGE_LOOP ( 'NONE', ( #6973, #1906 ) ) ;
#7451=VERTEX_POINT ( 'NONE', #3257 ) ;
#7458=DIRECTION ( 'NONE',  ( -0.000000000000000000, -0.000000000000000000, 1.000000000000000000 ) ) ;
#7461=DIRECTION ( 'NONE',  ( -0.000000000000000000, -0.000000000000000000, 1.000000000000000000 ) ) ;
#7476=DIRECTION ( 'NONE',  ( -0.000000000000000000, -0.000000000000000000, 1.000000000000000000 ) ) ;
#7482=AXIS2_PLACEMENT_3D ( 'NONE', #2494, #4882, #451 ) ;
#7492=EDGE_CURVE ( 'NONE', #984, #4671, #7279, .T. ) ;
#7508=DIRECTION ( 'NONE',  ( -1.000000000000000000, 0.000000000000000000, 0.000000000000000000 ) ) ;
#7517=DIRECTION ( 'NONE',  ( -1.000000000000000000, 0.000000000000000000, 0.000000000000000000 ) ) ;
#7534=DIRECTION ( 'NONE',  ( 1.460819769243626145E-16, -1.000000000000000000, 0.000000000000000000 ) ) ;
#7541=VERTEX_POINT ( 'NONE', #4739 ) ;
#7557=CARTESIAN_POINT ( 'NONE',  ( 115.0000000000000284, -115.0000000000000000, 20.00000000000000355 ) ) ;
#7560=CARTESIAN_POINT ( 'NONE',  ( 115.0000000000000284, -115.0000000000000000, 70.00000000000000000 ) ) ;
#7565=CARTESIAN_POINT ( 'NONE',  ( 121.0000000000000000, 115.0000000000000000, 70.00000000000000000 ) ) ;
#7567=CARTESIAN_POINT ( 'NONE',  ( 0.000000000000000000, 0.000000000000000000, 35.00000000000000000 ) ) ;
#7586=LINE ( 'NONE', #2443, #6014 ) ;
#7611=ORIENTED_EDGE ( 'NONE', *, *, #3991, .F. ) ;
#7615=ORIENTED_EDGE ( 'NONE', *, *, #3533, .F. ) ;
#7621=EDGE_LOOP ( 'NONE', ( #5478, #6921, #5591, #4369 ) ) ;
#7629=FACE_OUTER_BOUND ( 'NONE', #4275, .T. ) ;
#7632=LINE ( 'NONE', #4441, #1569 ) ;
#7638=CARTESIAN_POINT ( 'NONE',  ( -115.0000000000000000, 115.0000000000000000, 20.00000000000000355 ) ) ;
#7644=CARTESIAN_POINT ( 'NONE',  ( 125.0000000000000000, 125.0000000000000284, 70.00000000000000000 ) ) ;
#7645=CIRCLE ( 'NONE', #338, 75.00000000000001421 ) ;
#7652=EDGE_CURVE ( 'NONE', #4172, #6494, #1162, .T. ) ;
#7655=LINE ( 'NONE', #6367, #6165 ) ;
#7661=DIRECTION ( 'NONE',  ( -1.000000000000000000, 0.000000000000000000, -0.000000000000000000 ) ) ;
#7674=CARTESIAN_POINT ( 'NONE',  ( -125.0000000000000000, -125.0000000000000284, 70.00000000000000000 ) ) ;
#7683=ORIENTED_EDGE ( 'NONE', *, *, #3809, .T. ) ;
#7685=CARTESIAN_POINT ( 'NONE',  ( -125.0000000000000000, -125.0000000000000284, 70.00000000000000000 ) ) ;
#7686=EDGE_CURVE ( 'NONE', #431, #4314, #520, .T. ) ;
#7705=CARTESIAN_POINT ( 'NONE',  ( 0.000000000000000000, 0.000000000000000000, 0.000000000000000000 ) ) ;
#7711=CARTESIAN_POINT ( 'NONE',  ( 95.00000000000008527, 0.000000000000000000, 20.00000000000000355 ) ) ;
#7721=EDGE_LOOP ( 'NONE', ( #6454, #2547, #3519, #1768 ) ) ;
#7746=ORIENTED_EDGE ( 'NONE', *, *, #3375, .F. ) ;
#7765=DIRECTION ( 'NONE',  ( 1.000000000000000000, 0.000000000000000000, 0.000000000000000000 ) ) ;
#7773=CARTESIAN_POINT ( 'NONE',  ( -121.0000000000000000, 115.0000000000000000, 20.00000000000000355 ) ) ;
#7775=DIRECTION ( 'NONE',  ( 1.000000000000000000, 0.000000000000000000, 0.000000000000000000 ) ) ;
#7777=DIRECTION ( 'NONE',  ( 1.000000000000000000, 0.000000000000000000, 0.000000000000000000 ) ) ;
#7781=CIRCLE ( 'NONE', #6133, 75.00000000000001421 ) ;
#7793=DIRECTION ( 'NONE',  ( -1.000000000000000000, 0.000000000000000000, 0.000000000000000000 ) ) ;
#7801=VECTOR ( 'NONE', #704, 1000.000000000000000 ) ;
#7802=DIRECTION ( 'NONE',  ( -0.000000000000000000, -0.000000000000000000, -1.000000000000000000 ) ) ;
#7815=FACE_OUTER_BOUND ( 'NONE', #4221, .T. ) ;
#7816=ORIENTED_EDGE ( 'NONE', *, *, #3763, .T. ) ;
#7821=EDGE_CURVE ( 'NONE', #321, #4413, #4, .T. ) ;
#7824=EDGE_LOOP ( 'NONE', ( #3567, #405, #631, #7816 ) ) ;
#7828=VERTEX_POINT ( 'NONE', #7226 ) ;
#7838=CARTESIAN_POINT ( 'NONE',  ( 125.0000000000000000, 125.0000000000000284, 0.000000000000000000 ) ) ;
#7845=CARTESIAN_POINT ( 'NONE',  ( -121.0000000000000000, 115.0000000000000000, 70.00000000000000000 ) ) ;
#7852=EDGE_LOOP ( 'NONE', ( #7141, #3834 ) ) ;
#7869=DIRECTION ( 'NONE',  ( -0.8571673007021112234, 1.049727191138617340E-16, 0.5150380749100560429 ) ) ;
#7880=PLANE ( 'NONE',  #2010 ) ;
#7896=EDGE_CURVE ( 'NONE', #5876, #6392, #647, .T. ) ;
#7903=DIRECTION ( 'NONE',  ( -0.000000000000000000, -0.000000000000000000, 1.000000000000000000 ) ) ;
#7934=VERTEX_POINT ( 'NONE', #3326 ) ;
#7950=ORIENTED_EDGE ( 'NONE', *, *, #31, .F. ) ;
#7954=DIRECTION ( 'NONE',  ( 0.000000000000000000, 0.000000000000000000, -1.000000000000000000 ) ) ;
#7964=DIRECTION ( 'NONE',  ( 1.000000000000000000, 0.000000000000000000, 0.000000000000000000 ) ) ;
#7979=DIRECTION ( 'NONE',  ( -0.000000000000000000, -0.000000000000000000, 1.000000000000000000 ) ) ;
#7983=CARTESIAN_POINT ( 'NONE',  ( 0.000000000000000000, 0.000000000000000000, 35.00000000000000000 ) ) ;
#7988=VERTEX_POINT ( 'NONE', #6828 ) ;
#7999=DIRECTION ( 'NONE',  ( -0.000000000000000000, -0.000000000000000000, -1.000000000000000000 ) ) ;
#8009=EDGE_CURVE ( 'NONE', #4086, #2906, #4766, .T. ) ;
#8018=ORIENTED_EDGE ( 'NONE', *, *, #1346, .T. ) ;
#8019=CARTESIAN_POINT ( 'NONE',  ( 95.00000000000002842, -95.00000000000002842, 70.00000000000000000 ) ) ;
#8028=DIRECTION ( 'NONE',  ( -1.000000000000000000, 0.000000000000000000, -0.000000000000000000 ) ) ;
#8031=ADVANCED_FACE ( 'NONE', ( #3067 ), #5365, .F. ) ;
#8033=( NAMED_UNIT ( * ) PLANE_ANGLE_UNIT ( ) SI_UNIT ( $, .RADIAN. ) );
#8038=CYLINDRICAL_SURFACE ( 'NONE', #6498, 5.999999999999991118 ) ;
#8042=CARTESIAN_POINT ( 'NONE',  ( 121.0000000000000000, 115.0000000000000000, 70.00000000000000000 ) ) ;
#8062=AXIS2_PLACEMENT_3D ( 'NONE', #5919, #4009, #128 ) ;
#8069=DIRECTION ( 'NONE',  ( -0.000000000000000000, -0.000000000000000000, 1.000000000000000000 ) ) ;
#8075=APPLICATION_CONTEXT ( 'automotive_design' ) ;
#8081=CARTESIAN_POINT ( 'NONE',  ( 0.000000000000000000, 0.000000000000000000, 20.00000000000000355 ) ) ;
#8095=EDGE_CURVE ( 'NONE', #5603, #5439, #1086, .T. ) ;
#8102=VECTOR ( 'NONE', #4456, 1000.000000000000000 ) ;
#8105=EDGE_CURVE ( 'NONE', #2961, #7369, #5053, .T. ) ;
#8114=CARTESIAN_POINT ( 'NONE',  ( 95.00000000000000000, 95.00000000000008527, 35.00000000000000000 ) ) ;
#8119=ORIENTED_EDGE ( 'NONE', *, *, #2723, .F. ) ;
#8122=DIRECTION ( 'NONE',  ( 1.000000000000000000, 0.000000000000000000, 0.000000000000000000 ) ) ;
#8136=FACE_BOUND ( 'NONE', #2469, .T. ) ;
#8138=CARTESIAN_POINT ( 'NONE',  ( 95.00000000000000000, 95.00000000000008527, 70.00000000000000000 ) ) ;
#8145=ADVANCED_FACE ( 'NONE', ( #1267 ), #1227, .F. ) ;
#8152=VERTEX_POINT ( 'NONE', #5781 ) ;
#8156=ORIENTED_EDGE ( 'NONE', *, *, #7686, .F. ) ;
#8157=EDGE_CURVE ( 'NONE', #3656, #5937, #7781, .T. ) ;
#8177=CARTESIAN_POINT ( 'NONE',  ( -115.0000000000000284, -115.0000000000000000, 20.00000000000000355 ) ) ;
#8200=VECTOR ( 'NONE', #7999, 1000.000000000000000 ) ;
#8208=EDGE_CURVE ( 'NONE', #6616, #3725, #7632, .T. ) ;
#8225=EDGE_CURVE ( 'NONE', #5937, #6480, #8267, .T. ) ;
#8227=ORIENTED_EDGE ( 'NONE', *, *, #3319, .T. ) ;
#8257=EDGE_CURVE ( 'NONE', #7369, #4413, #3823, .T. ) ;
#8264=DIRECTION ( 'NONE',  ( -1.000000000000000000, 0.000000000000000000, -0.000000000000000000 ) ) ;
#8267=LINE ( 'NONE', #6989, #1030 ) ;
#8287=CIRCLE ( 'NONE', #38, 95.00000000000008527 ) ;
#8289=ORIENTED_EDGE ( 'NONE', *, *, #1015, .T. ) ;
#8301=EDGE_CURVE ( 'NONE', #3725, #6102, #3855, .T. ) ;
#8318=DIRECTION ( 'NONE',  ( -1.000000000000000000, 0.000000000000000000, 0.000000000000000000 ) ) ;
#8328=CARTESIAN_POINT ( 'NONE',  ( 125.0000000000000000, -125.0000000000000284, 70.00000000000000000 ) ) ;
#8341=VERTEX_POINT ( 'NONE', #6473 ) ;
#8345=DIRECTION ( 'NONE',  ( 0.8571673007021112234, 0.000000000000000000, 0.5150380749100560429 ) ) ;
#8394=COLOUR_RGB('Grey',0.48,0.52,0.57);
#8395=FILL_AREA_STYLE_COLOUR('',#8394);
#8396=FILL_AREA_STYLE('',(#8395));
#8397=SURFACE_STYLE_FILL_AREA(#8396);
#8398=SURFACE_SIDE_STYLE('',(#8397));
#8399=SURFACE_STYLE_USAGE(.BOTH.,#8398);
#8400=PRESENTATION_STYLE_ASSIGNMENT((#8399));
ENDSEC;
END-ISO-10303-21;
